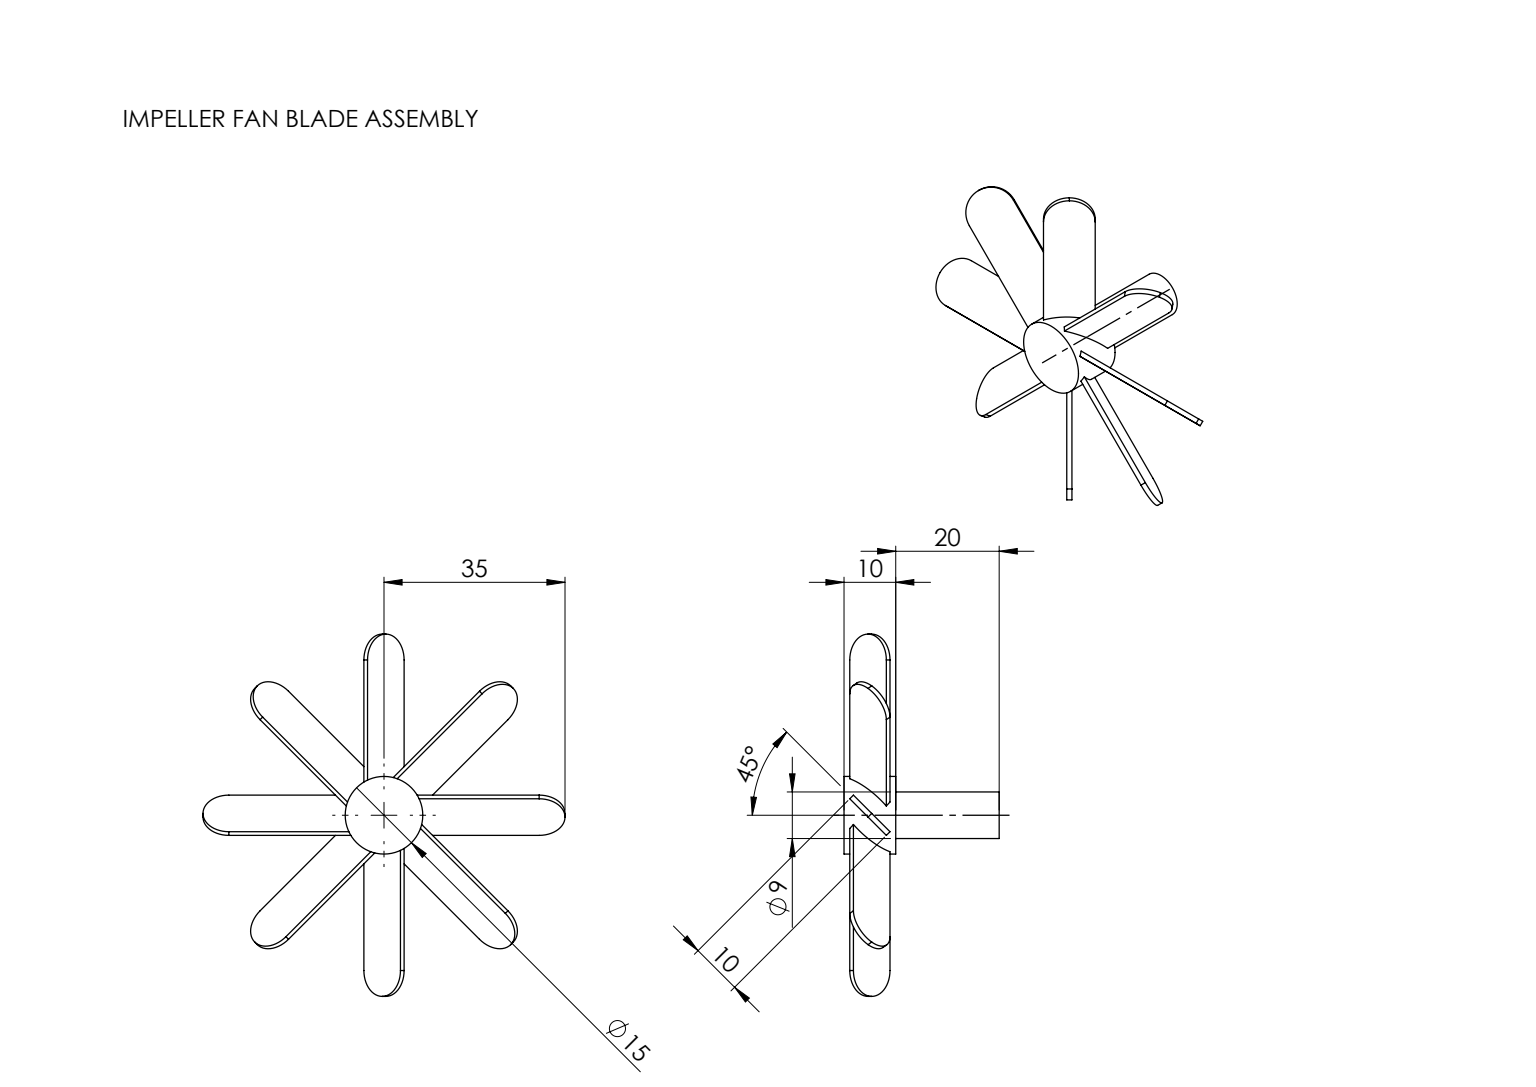
ISO-10303-21;
HEADER;
FILE_DESCRIPTION (('STEP AP214'),
    '1' );
FILE_NAME ('Impeller Fan Blade Assembly.step',
    '2026-10-04T13:31:42',
    ( '' ),
    ( '' ),
    'SwSTEP 2.0',
    'SolidWorks 2026',
    '' );
FILE_SCHEMA (( 'AUTOMOTIVE_DESIGN' ));
ENDSEC;

DATA;
#5=ORIENTED_EDGE ( 'NONE', *, *, #6876, .T. ) ;
#55=EDGE_CURVE ( 'NONE', #141361, #196966, #36036, .T. ) ;
#108=DIRECTION ( 'NONE',  ( -0.000000000000000000, -0.000000000000000000, -1.000000000000000000 ) ) ;
#589=CARTESIAN_POINT ( 'NONE',  ( -30.00000000000000355, 0.3535533905932703447, 5.353553390593268624 ) ) ;
#689=CARTESIAN_POINT ( 'NONE',  ( -3.181980515339399851, 6.791538853603101167, 8.889087296526001936 ) ) ;
#723=VERTEX_POINT ( 'NONE', #107411 ) ;
#910=CIRCLE ( 'NONE', #26805, 5.000000000000000000 ) ;
#1107=EDGE_CURVE ( 'NONE', #17186, #144635, #184276, .T. ) ;
#1119=DIRECTION ( 'NONE',  ( -0.8164965809277249242, 0.000000000000000000, 0.5773502691896271743 ) ) ;
#1198=AXIS2_PLACEMENT_3D ( 'NONE', #589, #95589, #143077 ) ;
#1251=( BOUNDED_CURVE ( )  B_SPLINE_CURVE ( 3, ( #125567, #152909, #47741, #154906 ),
 .UNSPECIFIED., .F., .T. ) 
 B_SPLINE_CURVE_WITH_KNOTS ( ( 4, 4 ),
 ( 2.008945357379067431, 2.115944711806982514 ),
 .UNSPECIFIED. ) 
 CURVE ( )  GEOMETRIC_REPRESENTATION_ITEM ( )  RATIONAL_B_SPLINE_CURVE ( ( 1.000000000000000000, 0.9990461557208837329, 0.9990461557208837329, 1.000000000000000000 ) ) 
 REPRESENTATION_ITEM ( '' )  );
#1322=FACE_OUTER_BOUND ( 'NONE', #192429, .T. ) ;
#1347=EDGE_CURVE ( 'NONE', #15917, #80087, #46585, .T. ) ;
#1367=CARTESIAN_POINT ( 'NONE',  ( 0.3535533905935857035, 30.00000000000000000, 5.353553390593269512 ) ) ;
#1528=CARTESIAN_POINT ( 'NONE',  ( 26.99873734152944138, 22.49873734152883387, 1.110912703473986074 ) ) ;
#1540=CIRCLE ( 'NONE', #59712, 5.000000000000000888 ) ;
#1624=AXIS2_PLACEMENT_3D ( 'NONE', #95423, #190434, #66079 ) ;
#1785=CARTESIAN_POINT ( 'NONE',  ( 4.500000000000000000, 0.000000000000000000, 0.000000000000000000 ) ) ;
#1856=ORIENTED_EDGE ( 'NONE', *, *, #13659, .T. ) ;
#1902=ORIENTED_EDGE ( 'NONE', *, *, #135350, .T. ) ;
#2136=DIRECTION ( 'NONE',  ( -0.7071067811865466846, 2.468850131082262583E-15, 0.7071067811865484609 ) ) ;
#2501=EDGE_CURVE ( 'NONE', #144635, #114656, #107792, .T. ) ;
#2531=DIRECTION ( 'NONE',  ( -0.7071067811865467956, 2.468850131082262977E-15, 0.7071067811865483499 ) ) ;
#2575=ADVANCED_FACE ( 'NONE', ( #39541 ), #193239, .T. ) ;
#2692=CARTESIAN_POINT ( 'NONE',  ( -3.660253528765552655, 6.551653823223177575, 8.410814283099849575 ) ) ;
#2908=DIRECTION ( 'NONE',  ( 0.8164965809277261455, 0.000000000000000000, 0.5773502691896257311 ) ) ;
#2998=CIRCLE ( 'NONE', #35325, 5.000000000000000000 ) ;
#3003=EDGE_CURVE ( 'NONE', #196688, #171715, #100113, .T. ) ;
#3105=EDGE_CURVE ( 'NONE', #165429, #128792, #7889, .T. ) ;
#3150=EDGE_CURVE ( 'NONE', #42832, #9747, #47569, .T. ) ;
#3534=FACE_OUTER_BOUND ( 'NONE', #60688, .T. ) ;
#3693=CARTESIAN_POINT ( 'NONE',  ( -21.99873734152892268, 27.49873734152935967, 1.818019484660534424 ) ) ;
#3699=LINE ( 'NONE', #80542, #50035 ) ;
#3706=CARTESIAN_POINT ( 'NONE',  ( 3.181980515339348337, -35.00000000000001421, 8.889087296526001936 ) ) ;
#3913=CARTESIAN_POINT ( 'NONE',  ( -7.500000000000000888, 1.380023386739105407, 4.327083394447439169 ) ) ;
#3974=PLANE ( 'NONE',  #72309 ) ;
#3984=DIRECTION ( 'NONE',  ( -0.7071067811865467956, 0.000000000000000000, 0.7071067811865483499 ) ) ;
#4050=DIRECTION ( 'NONE',  ( -1.047444401652940164E-14, -1.000000000000000000, -0.000000000000000000 ) ) ;
#4144=CARTESIAN_POINT ( 'NONE',  ( -6.412877669190335972, 3.889087296526014814, 1.818019484660534424 ) ) ;
#4246=VERTEX_POINT ( 'NONE', #76836 ) ;
#4281=CARTESIAN_POINT ( 'NONE',  ( -0.3535533905933930798, -35.00000000000000000, 5.353553390593270400 ) ) ;
#4343=CARTESIAN_POINT ( 'NONE',  ( -30.00000000000000355, 0.3535533905932729537, 5.353553390593267736 ) ) ;
#4363=CIRCLE ( 'NONE', #120577, 4.500000000000000000 ) ;
#4390=EDGE_LOOP ( 'NONE', ( #44839, #29813, #144030, #184763 ) ) ;
#4454=EDGE_CURVE ( 'NONE', #48994, #85047, #178636, .T. ) ;
#4626=VERTEX_POINT ( 'NONE', #89603 ) ;
#4692=ORIENTED_EDGE ( 'NONE', *, *, #3003, .F. ) ;
#4756=DIRECTION ( 'NONE',  ( -0.4999999999999967804, 0.5000000000000019984, 0.7071067811865484609 ) ) ;
#4830=VECTOR ( 'NONE', #8942, 1000.000000000000000 ) ;
#4878=VECTOR ( 'NONE', #141249, 1000.000000000000000 ) ;
#4970=FACE_OUTER_BOUND ( 'NONE', #19771, .T. ) ;
#5025=DIRECTION ( 'NONE',  ( -0.7071067811865466846, 7.406550393246786959E-15, -0.7071067811865484609 ) ) ;
#5159=DIRECTION ( 'NONE',  ( 0.5000000000000004441, 0.4999999999999987232, -0.7071067811865482389 ) ) ;
#5238=CARTESIAN_POINT ( 'NONE',  ( 3.660253528765602393, -6.551653823223149153, 8.410814283099844246 ) ) ;
#5316=CARTESIAN_POINT ( 'NONE',  ( 2.044528755335677683, -7.220908937440018605, 1.589185716900141321 ) ) ;
#5451=ORIENTED_EDGE ( 'NONE', *, *, #13659, .F. ) ;
#5503=CARTESIAN_POINT ( 'NONE',  ( 3.181980515339782212, 29.99999999999996803, 1.110912703473986074 ) ) ;
#5513=DIRECTION ( 'NONE',  ( 0.7071067811865414665, -0.7071067811865536790, -0.000000000000000000 ) ) ;
#5740=CARTESIAN_POINT ( 'NONE',  ( -21.99873734152930638, -27.49873734152905413, 8.181980515339454030 ) ) ;
#5918=CARTESIAN_POINT ( 'NONE',  ( -6.791538853603066528, 3.181980515339468241, 1.110912703473986074 ) ) ;
#5983=ORIENTED_EDGE ( 'NONE', *, *, #3150, .T. ) ;
#6136=AXIS2_PLACEMENT_3D ( 'NONE', #66629, #172837, #37289 ) ;
#6324=CARTESIAN_POINT ( 'NONE',  ( 35.00000000000000000, -3.181980515339468241, 1.110912703473986074 ) ) ;
#6392=ORIENTED_EDGE ( 'NONE', *, *, #134059, .T. ) ;
#6445=ORIENTED_EDGE ( 'NONE', *, *, #56848, .T. ) ;
#6595=VECTOR ( 'NONE', #69761, 1000.000000000000000 ) ;
#6659=CARTESIAN_POINT ( 'NONE',  ( -23.96320343559627375, 18.46320343559663257, 8.181980515339452253 ) ) ;
#6681=VERTEX_POINT ( 'NONE', #26746 ) ;
#6876=EDGE_CURVE ( 'NONE', #157949, #129810, #101294, .T. ) ;
#6906=EDGE_CURVE ( 'NONE', #84463, #144635, #114277, .T. ) ;
#7056=CARTESIAN_POINT ( 'NONE',  ( -3.181980515339590365, -34.99999999999999289, 1.110912703473986074 ) ) ;
#7236=CARTESIAN_POINT ( 'NONE',  ( 3.889087296525994830, -6.412877669190346630, 8.181980515339454030 ) ) ;
#7349=ADVANCED_FACE ( 'NONE', ( #109514 ), #171196, .T. ) ;
#7427=DIRECTION ( 'NONE',  ( 0.7071067811865483499, 0.000000000000000000, -0.7071067811865465735 ) ) ;
#7479=ORIENTED_EDGE ( 'NONE', *, *, #86511, .F. ) ;
#7567=CARTESIAN_POINT ( 'NONE',  ( 3.181980515339834614, 34.99999999999997158, 1.110912703473986074 ) ) ;
#7576=ORIENTED_EDGE ( 'NONE', *, *, #27260, .F. ) ;
#7667=LINE ( 'NONE', #113841, #95061 ) ;
#7672=PLANE ( 'NONE',  #93602 ) ;
#7889=CIRCLE ( 'NONE', #130564, 5.000000000000000000 ) ;
#7900=STYLED_ITEM ( 'NONE', ( #152730 ), #117169 ) ;
#8055=ORIENTED_EDGE ( 'NONE', *, *, #1107, .F. ) ;
#8138=EDGE_CURVE ( 'NONE', #13627, #4626, #1540, .T. ) ;
#8335=SHAPE_REPRESENTATION ( 'Impeller Fan Blade Assembly', ( #82054 ), #65912 ) ;
#8564=DIRECTION ( 'NONE',  ( 0.000000000000000000, -0.7071067811865483499, -0.7071067811865467956 ) ) ;
#8687=CARTESIAN_POINT ( 'NONE',  ( -30.00000000000000355, -0.3535533905932729537, 4.646446609406719830 ) ) ;
#8817=CIRCLE ( 'NONE', #41014, 4.999999999999999112 ) ;
#8942=DIRECTION ( 'NONE',  ( -0.7071067811865561215, -0.7071067811865389130, -0.000000000000000000 ) ) ;
#8948=ADVANCED_FACE ( 'NONE', ( #56337 ), #72517, .T. ) ;
#9057=CARTESIAN_POINT ( 'NONE',  ( 1.784589286804253661, -7.284589286804279418, 1.818019484660534424 ) ) ;
#9330=CARTESIAN_POINT ( 'NONE',  ( 4.500000000000000000, 0.000000000000000000, -20.00000000000000000 ) ) ;
#9490=DIRECTION ( 'NONE',  ( -0.7071067811865483499, 7.406550393246807469E-15, 0.7071067811865467956 ) ) ;
#9504=DIRECTION ( 'NONE',  ( -0.4999999999999966693, 0.5000000000000019984, 0.7071067811865484609 ) ) ;
#9508=VERTEX_POINT ( 'NONE', #142115 ) ;
#9572=CARTESIAN_POINT ( 'NONE',  ( 20.96320343559639454, -21.46320343559646560, 5.353553390593268624 ) ) ;
#9574=CARTESIAN_POINT ( 'NONE',  ( 6.791538853603070081, -3.181980515339468241, 1.110912703473986074 ) ) ;
#9721=ORIENTED_EDGE ( 'NONE', *, *, #167487, .T. ) ;
#9747=VERTEX_POINT ( 'NONE', #90410 ) ;
#10026=CARTESIAN_POINT ( 'NONE',  ( 7.500000000000000000, 9.184850993605147944E-16, 10.00000000000000000 ) ) ;
#10163=DIRECTION ( 'NONE',  ( 3.491481338843133750E-15, 1.000000000000000000, -0.000000000000000000 ) ) ;
#10280=EDGE_CURVE ( 'NONE', #27947, #199067, #69380, .T. ) ;
#10292=AXIS2_PLACEMENT_3D ( 'NONE', #91072, #108246, #169925 ) ;
#10463=DIRECTION ( 'NONE',  ( 3.491481338843133750E-15, 1.000000000000000000, -0.000000000000000000 ) ) ;
#10721=EDGE_LOOP ( 'NONE', ( #25511, #113334, #196537, #77150 ) ) ;
#10785=DIRECTION ( 'NONE',  ( -0.5000000000000004441, -0.4999999999999986122, 0.7071067811865481278 ) ) ;
#10842=EDGE_CURVE ( 'NONE', #178298, #133752, #105049, .T. ) ;
#11040=ORIENTED_EDGE ( 'NONE', *, *, #91376, .T. ) ;
#11092=CIRCLE ( 'NONE', #108041, 5.000000000000000888 ) ;
#11219=ADVANCED_FACE ( 'NONE', ( #166041 ), #39684, .T. ) ;
#11295=DIRECTION ( 'NONE',  ( 0.000000000000000000, 0.000000000000000000, -1.000000000000000000 ) ) ;
#11355=LINE ( 'NONE', #146847, #59682 ) ;
#11514=PLANE ( 'NONE',  #138109 ) ;
#11543=EDGE_LOOP ( 'NONE', ( #139060, #54030, #101271, #76583, #175395 ) ) ;
#11617=ORIENTED_EDGE ( 'NONE', *, *, #69929, .F. ) ;
#11630=AXIS2_PLACEMENT_3D ( 'NONE', #120508, #167033, #180236 ) ;
#11743=CARTESIAN_POINT ( 'NONE',  ( 1.784589286804354247, 7.284589286804251884, 8.181980515339454030 ) ) ;
#11932=( BOUNDED_CURVE ( )  B_SPLINE_CURVE ( 3, ( #178851, #190018, #191005, #82807 ),
 .UNSPECIFIED., .F., .T. ) 
 B_SPLINE_CURVE_WITH_KNOTS ( ( 4, 4 ),
 ( 1.570796326794896780, 2.008945357379067875 ),
 .UNSPECIFIED. ) 
 CURVE ( )  GEOMETRIC_REPRESENTATION_ITEM ( )  RATIONAL_B_SPLINE_CURVE ( ( 1.000000000000000000, 0.9840659996946589105, 0.9840659996946589105, 1.000000000000000000 ) ) 
 REPRESENTATION_ITEM ( '' )  );
#12043=ORIENTED_EDGE ( 'NONE', *, *, #15456, .T. ) ;
#12294=DIRECTION ( 'NONE',  ( 0.7071067811865483499, 0.000000000000000000, 0.7071067811865465735 ) ) ;
#12421=ORIENTED_EDGE ( 'NONE', *, *, #88897, .T. ) ;
#12432=EDGE_CURVE ( 'NONE', #166399, #177515, #11092, .T. ) ;
#12454=LINE ( 'NONE', #42781, #99287 ) ;
#12531=EDGE_LOOP ( 'NONE', ( #95723, #112577, #18902, #136968, #137957 ) ) ;
#12569=CARTESIAN_POINT ( 'NONE',  ( 3.889087296526082316, 6.412877669190294228, 1.818019484660534424 ) ) ;
#12967=ADVANCED_FACE ( 'NONE', ( #39608 ), #101267, .T. ) ;
#13016=EDGE_LOOP ( 'NONE', ( #106007, #37558 ) ) ;
#13023=EDGE_LOOP ( 'NONE', ( #163707, #150234, #31137, #136726 ) ) ;
#13033=ORIENTED_EDGE ( 'NONE', *, *, #147612, .T. ) ;
#13111=EDGE_CURVE ( 'NONE', #198713, #191800, #40221, .T. ) ;
#13247=SURFACE_SIDE_STYLE ('',( #59729 ) ) ;
#13272=CARTESIAN_POINT ( 'NONE',  ( -0.3535533905933784249, -30.00000000000000000, 5.353553390593268624 ) ) ;
#13320=EDGE_CURVE ( 'NONE', #81477, #29557, #156408, .T. ) ;
#13428=CARTESIAN_POINT ( 'NONE',  ( -3.889087296526120063, -29.99999999999998579, 1.818019484660534424 ) ) ;
#13627=VERTEX_POINT ( 'NONE', #119460 ) ;
#13659=EDGE_CURVE ( 'NONE', #42657, #30159, #117744, .T. ) ;
#13686=EDGE_LOOP ( 'NONE', ( #100957, #99162, #122870, #78497, #107366, #112026 ) ) ;
#13931=CARTESIAN_POINT ( 'NONE',  ( -2.044528755335630166, 7.220908937440031039, 1.589185716900140211 ) ) ;
#14009=CARTESIAN_POINT ( 'NONE',  ( -18.46320343559655086, -23.96320343559633059, 8.181980515339455806 ) ) ;
#14059=LINE ( 'NONE', #26274, #159692 ) ;
#14195=EDGE_CURVE ( 'NONE', #96881, #9508, #7667, .T. ) ;
#14313=VECTOR ( 'NONE', #102691, 1000.000000000000114 ) ;
#14408=DIRECTION ( 'NONE',  ( 0.000000000000000000, 0.7071067811865467956, -0.7071067811865483499 ) ) ;
#14414=LINE ( 'NONE', #123563, #33888 ) ;
#14524=CIRCLE ( 'NONE', #82328, 5.000000000000000888 ) ;
#14739=CARTESIAN_POINT ( 'NONE',  ( -7.220908937440027486, -2.044528755335643044, 1.589185716900149092 ) ) ;
#14812=ORIENTED_EDGE ( 'NONE', *, *, #128355, .F. ) ;
#14925=DIRECTION ( 'NONE',  ( 0.5000000000000037748, 0.4999999999999950595, 0.7071067811865484609 ) ) ;
#15121=CARTESIAN_POINT ( 'NONE',  ( -30.00000000000000355, -3.889087296526017479, 8.181980515339454030 ) ) ;
#15152=VECTOR ( 'NONE', #148657, 1000.000000000000000 ) ;
#15282=VECTOR ( 'NONE', #95551, 1000.000000000000000 ) ;
#15456=EDGE_CURVE ( 'NONE', #9747, #199879, #95459, .T. ) ;
#15553=CARTESIAN_POINT ( 'NONE',  ( 30.00000000000000355, -3.889087296526015258, 1.818019484660534646 ) ) ;
#15917=VERTEX_POINT ( 'NONE', #99441 ) ;
#15975=CIRCLE ( 'NONE', #116131, 5.000000000000000000 ) ;
#16098=LINE ( 'NONE', #64586, #153351 ) ;
#16296=DIRECTION ( 'NONE',  ( -1.000000000000000000, 0.000000000000000000, 0.000000000000000000 ) ) ;
#16411=CARTESIAN_POINT ( 'NONE',  ( -2.552343178074661267, -7.052343178074616858, 8.889087296526001936 ) ) ;
#16715=DIRECTION ( 'NONE',  ( 0.5000000000000014433, 0.4999999999999996114, 0.7071067811865467956 ) ) ;
#16726=CARTESIAN_POINT ( 'NONE',  ( 6.791538853603062975, 3.181980515339470905, 8.889087296526001936 ) ) ;
#16796=ORIENTED_EDGE ( 'NONE', *, *, #105651, .T. ) ;
#16838=EDGE_CURVE ( 'NONE', #172390, #19226, #143704, .T. ) ;
#16899=CARTESIAN_POINT ( 'NONE',  ( 6.412877669190335972, -3.889087296526014814, 1.818019484660534424 ) ) ;
#17186=VERTEX_POINT ( 'NONE', #124573 ) ;
#17220=ORIENTED_EDGE ( 'NONE', *, *, #112155, .T. ) ;
#17363=VERTEX_POINT ( 'NONE', #16411 ) ;
#17418=EDGE_CURVE ( 'NONE', #75343, #15917, #153385, .T. ) ;
#17615=EDGE_CURVE ( 'NONE', #85047, #60651, #14414, .T. ) ;
#17635=DIRECTION ( 'NONE',  ( -0.000000000000000000, -0.000000000000000000, -1.000000000000000000 ) ) ;
#17870=AXIS2_PLACEMENT_3D ( 'NONE', #4343, #130687, #157056 ) ;
#17909=ORIENTED_EDGE ( 'NONE', *, *, #89293, .T. ) ;
#17930=DIRECTION ( 'NONE',  ( 0.000000000000000000, -0.7071067811865467956, -0.7071067811865483499 ) ) ;
#18096=CARTESIAN_POINT ( 'NONE',  ( -7.284589286804255437, 1.784589286804319386, 8.181980515339454030 ) ) ;
#18224=VERTEX_POINT ( 'NONE', #160889 ) ;
#18467=VECTOR ( 'NONE', #74443, 1000.000000000000000 ) ;
#18598=ORIENTED_EDGE ( 'NONE', *, *, #48667, .F. ) ;
#18660=ORIENTED_EDGE ( 'NONE', *, *, #193497, .T. ) ;
#18750=AXIS2_PLACEMENT_3D ( 'NONE', #120314, #42501, #61612 ) ;
#18902=ORIENTED_EDGE ( 'NONE', *, *, #136231, .T. ) ;
#18906=EDGE_CURVE ( 'NONE', #96881, #27352, #98517, .T. ) ;
#19107=CARTESIAN_POINT ( 'NONE',  ( -7.128481858827110607, 2.709097808555396281, 2.998008972631150737 ) ) ;
#19109=DIRECTION ( 'NONE',  ( 0.7071067811865483499, -2.468850131082268499E-15, 0.7071067811865467956 ) ) ;
#19226=VERTEX_POINT ( 'NONE', #185021 ) ;
#19309=CARTESIAN_POINT ( 'NONE',  ( -3.181980515339399851, 6.791538853603101167, 8.889087296526001936 ) ) ;
#19710=DIRECTION ( 'NONE',  ( 0.000000000000000000, -0.8164965809277239250, -0.5773502691896288397 ) ) ;
#19771=EDGE_LOOP ( 'NONE', ( #190197, #68449, #74086, #157970 ) ) ;
#19850=CARTESIAN_POINT ( 'NONE',  ( -3.424326230466266718, 6.677994727576254341, 8.646741581399135512 ) ) ;
#19925=ADVANCED_FACE ( 'NONE', ( #188018 ), #156674, .T. ) ;
#19960=EDGE_LOOP ( 'NONE', ( #159693, #6392, #38372, #30787 ) ) ;
#20100=PLANE ( 'NONE',  #147708 ) ;
#20134=CARTESIAN_POINT ( 'NONE',  ( 0.3535533905935844268, 30.00000000000000000, 5.353553390593268624 ) ) ;
#20188=ORIENTED_EDGE ( 'NONE', *, *, #57355, .T. ) ;
#20191=DIRECTION ( 'NONE',  ( -0.4999999999999966693, 0.5000000000000019984, 0.7071067811865483499 ) ) ;
#20248=EDGE_CURVE ( 'NONE', #178298, #138583, #149478, .T. ) ;
#20336=DIRECTION ( 'NONE',  ( 0.5000000000000037748, 0.4999999999999950040, 0.7071067811865484609 ) ) ;
#20570=VERTEX_POINT ( 'NONE', #197973 ) ;
#20607=DIRECTION ( 'NONE',  ( 1.000000000000000000, 0.000000000000000000, -0.000000000000000000 ) ) ;
#20686=ORIENTED_EDGE ( 'NONE', *, *, #10842, .T. ) ;
#20694=CARTESIAN_POINT ( 'NONE',  ( -22.49873734152930282, -26.99873734152905058, 8.889087296526001936 ) ) ;
#20858=CARTESIAN_POINT ( 'NONE',  ( 3.181980515339539295, 6.791538853603031889, 1.110912703473986074 ) ) ;
#20991=VECTOR ( 'NONE', #68552, 1000.000000000000000 ) ;
#21095=CARTESIAN_POINT ( 'NONE',  ( -7.500000000000000000, 0.000000000000000000, 4.292893218813445877 ) ) ;
#21117=LINE ( 'NONE', #174809, #43151 ) ;
#21147=VECTOR ( 'NONE', #98013, 1000.000000000000000 ) ;
#21379=DIRECTION ( 'NONE',  ( 0.000000000000000000, 0.8164965809277239250, 0.5773502691896288397 ) ) ;
#21384=VECTOR ( 'NONE', #104477, 1000.000000000000000 ) ;
#21394=ORIENTED_EDGE ( 'NONE', *, *, #126396, .T. ) ;
#21707=CARTESIAN_POINT ( 'NONE',  ( 27.49873734152913229, -21.99873734152921045, 8.181980515339454030 ) ) ;
#21733=FACE_OUTER_BOUND ( 'NONE', #88711, .T. ) ;
#21856=DIRECTION ( 'NONE',  ( 1.000000000000000000, -0.000000000000000000, -0.000000000000000000 ) ) ;
#22083=CARTESIAN_POINT ( 'NONE',  ( -6.412877669190335972, 3.889087296526014814, 1.818019484660534424 ) ) ;
#22192=ORIENTED_EDGE ( 'NONE', *, *, #13320, .T. ) ;
#22226=DIRECTION ( 'NONE',  ( 1.000000000000000000, -0.000000000000000000, -0.000000000000000000 ) ) ;
#22425=CARTESIAN_POINT ( 'NONE',  ( 3.181980515339446924, -6.791538853603077186, 8.889087296526001936 ) ) ;
#22619=PLANE ( 'NONE',  #91802 ) ;
#22670=EDGE_LOOP ( 'NONE', ( #127996, #170160, #88143, #37570 ) ) ;
#22862=CARTESIAN_POINT ( 'NONE',  ( -22.49873734152892624, 26.99873734152936677, 1.110912703473986074 ) ) ;
#22871=DIRECTION ( 'NONE',  ( -0.5000000000000037748, -0.4999999999999950595, -0.7071067811865484609 ) ) ;
#23387=CARTESIAN_POINT ( 'NONE',  ( -7.500000000000000000, 0.000000000000000000, 5.707106781186540800 ) ) ;
#23431=ORIENTED_EDGE ( 'NONE', *, *, #100813, .F. ) ;
#23455=ORIENTED_EDGE ( 'NONE', *, *, #67374, .T. ) ;
#23492=DIRECTION ( 'NONE',  ( -0.5000000000000037748, -0.4999999999999950595, -0.7071067811865484609 ) ) ;
#23611=VERTEX_POINT ( 'NONE', #176579 ) ;
#23632=CARTESIAN_POINT ( 'NONE',  ( -7.052343178074620411, 2.552343178074692354, 8.889087296526001936 ) ) ;
#23740=CARTESIAN_POINT ( 'NONE',  ( 3.660253528765689435, 6.551653823223101192, 1.589185716900141543 ) ) ;
#23852=DIRECTION ( 'NONE',  ( -0.000000000000000000, 0.7071067811865466846, -0.7071067811865484609 ) ) ;
#23886=AXIS2_PLACEMENT_3D ( 'NONE', #181840, #166675, #55488 ) ;
#24008=ORIENTED_EDGE ( 'NONE', *, *, #133545, .T. ) ;
#24394=DIRECTION ( 'NONE',  ( 0.000000000000000000, -0.7071067811865485719, 0.7071067811865465735 ) ) ;
#24399=CARTESIAN_POINT ( 'NONE',  ( -26.99873734152928506, -22.49873734152901861, 1.110912703473986074 ) ) ;
#24590=ORIENTED_EDGE ( 'NONE', *, *, #123454, .T. ) ;
#24593=ORIENTED_EDGE ( 'NONE', *, *, #170916, .F. ) ;
#24595=ORIENTED_EDGE ( 'NONE', *, *, #145326, .F. ) ;
#24627=CARTESIAN_POINT ( 'NONE',  ( 21.99873734152949822, 27.49873734152890137, 8.181980515339454030 ) ) ;
#24679=CYLINDRICAL_SURFACE ( 'NONE', #186623, 5.000000000000002665 ) ;
#24832=ORIENTED_EDGE ( 'NONE', *, *, #149135, .T. ) ;
#25131=ORIENTED_EDGE ( 'NONE', *, *, #52643, .F. ) ;
#25203=CARTESIAN_POINT ( 'NONE',  ( 20.96320343559668942, 21.46320343559617427, 4.646446609406718942 ) ) ;
#25449=EDGE_CURVE ( 'NONE', #144525, #33153, #188245, .T. ) ;
#25474=CARTESIAN_POINT ( 'NONE',  ( 0.000000000000000000, 0.000000000000000000, 0.000000000000000000 ) ) ;
#25511=ORIENTED_EDGE ( 'NONE', *, *, #129609, .F. ) ;
#25535=CARTESIAN_POINT ( 'NONE',  ( 2.552343178074723884, 7.052343178074616858, 8.889087296526001936 ) ) ;
#25754=CARTESIAN_POINT ( 'NONE',  ( 6.551653823223139383, -3.660253528765621045, 1.589185716900141543 ) ) ;
#25888=ORIENTED_EDGE ( 'NONE', *, *, #28343, .F. ) ;
#26096=( BOUNDED_CURVE ( )  B_SPLINE_CURVE ( 3, ( #116778, #194637, #103622, #42945 ),
 .UNSPECIFIED., .F., .T. ) 
 B_SPLINE_CURVE_WITH_KNOTS ( ( 4, 4 ),
 ( 1.132647296210726795, 2.115944711806982514 ),
 .UNSPECIFIED. ) 
 CURVE ( )  GEOMETRIC_REPRESENTATION_ITEM ( )  RATIONAL_B_SPLINE_CURVE ( ( 1.000000000000000000, 0.9210371567966664230, 0.9210371567966664230, 1.000000000000000000 ) ) 
 REPRESENTATION_ITEM ( '' )  );
#26126=VERTEX_POINT ( 'NONE', #40621 ) ;
#26274=CARTESIAN_POINT ( 'NONE',  ( 3.889087296525912674, -30.00000000000002132, 8.181980515339454030 ) ) ;
#26660=CARTESIAN_POINT ( 'NONE',  ( -3.181980515339104532, 35.00000000000003553, 8.889087296526001936 ) ) ;
#26746=CARTESIAN_POINT ( 'NONE',  ( -30.00000000000000355, -3.181980515339470905, 8.889087296526001936 ) ) ;
#26791=CARTESIAN_POINT ( 'NONE',  ( 3.889087296526381632, 34.99999999999996447, 1.818019484660534424 ) ) ;
#26805=AXIS2_PLACEMENT_3D ( 'NONE', #91589, #92593, #153279 ) ;
#26877=CARTESIAN_POINT ( 'NONE',  ( -4.500000000000000000, 5.510910596163088569E-16, -20.00000000000000000 ) ) ;
#26894=VERTEX_POINT ( 'NONE', #49568 ) ;
#27082=AXIS2_PLACEMENT_3D ( 'NONE', #20694, #84353, #19710 ) ;
#27260=EDGE_CURVE ( 'NONE', #90645, #95772, #139430, .T. ) ;
#27280=MECHANICAL_DESIGN_GEOMETRIC_PRESENTATION_REPRESENTATION('',(#7900),#130572);
#27352=VERTEX_POINT ( 'NONE', #184110 ) ;
#27375=ORIENTED_EDGE ( 'NONE', *, *, #136231, .F. ) ;
#27439=EDGE_LOOP ( 'NONE', ( #5, #177531, #143908, #11617 ) ) ;
#27493=AXIS2_PLACEMENT_3D ( 'NONE', #111358, #20336, #63870 ) ;
#27596=ORIENTED_EDGE ( 'NONE', *, *, #126710, .F. ) ;
#27682=CARTESIAN_POINT ( 'NONE',  ( 21.46320343559668231, 20.96320343559617072, 5.353553390593268624 ) ) ;
#27947=VERTEX_POINT ( 'NONE', #144552 ) ;
#28043=EDGE_CURVE ( 'NONE', #60651, #37524, #38130, .T. ) ;
#28210=ADVANCED_FACE ( 'NONE', ( #138111 ), #87873, .F. ) ;
#28306=VERTEX_POINT ( 'NONE', #162728 ) ;
#28321=CARTESIAN_POINT ( 'NONE',  ( 35.00000000000000000, -0.3535533905932707888, 5.353553390593270400 ) ) ;
#28343=EDGE_CURVE ( 'NONE', #37524, #123075, #155634, .T. ) ;
#28437=VERTEX_POINT ( 'NONE', #85884 ) ;
#28509=CYLINDRICAL_SURFACE ( 'NONE', #190488, 7.500000000000000000 ) ;
#28733=DIRECTION ( 'NONE',  ( -0.5000000000000004441, -0.4999999999999987232, 0.7071067811865482389 ) ) ;
#29121=AXIS2_PLACEMENT_3D ( 'NONE', #119864, #43028, #90504 ) ;
#29203=CARTESIAN_POINT ( 'NONE',  ( 35.00000000000000000, -3.181980515339468241, 1.110912703473986074 ) ) ;
#29290=VECTOR ( 'NONE', #123695, 1000.000000000000000 ) ;
#29437=DIRECTION ( 'NONE',  ( 0.000000000000000000, 0.000000000000000000, -1.000000000000000000 ) ) ;
#29441=EDGE_LOOP ( 'NONE', ( #71166, #121903, #199643, #195876, #16796, #178830 ) ) ;
#29557=VERTEX_POINT ( 'NONE', #181399 ) ;
#29584=CARTESIAN_POINT ( 'NONE',  ( -6.791538853603066528, -3.181980515339470905, 8.889087296526001936 ) ) ;
#29707=DIRECTION ( 'NONE',  ( -0.000000000000000000, -0.7071067811865467956, 0.7071067811865483499 ) ) ;
#29813=ORIENTED_EDGE ( 'NONE', *, *, #165696, .T. ) ;
#30159=VERTEX_POINT ( 'NONE', #4281 ) ;
#30610=CYLINDRICAL_SURFACE ( 'NONE', #50415, 5.000000000000000000 ) ;
#30636=VERTEX_POINT ( 'NONE', #44613 ) ;
#30664=ORIENTED_EDGE ( 'NONE', *, *, #41288, .F. ) ;
#30694=DIRECTION ( 'NONE',  ( 0.000000000000000000, -0.7071067811865467956, 0.7071067811865483499 ) ) ;
#30703=CARTESIAN_POINT ( 'NONE',  ( 24.49873734152946625, 24.99873734152886939, 4.646446609406719830 ) ) ;
#30787=ORIENTED_EDGE ( 'NONE', *, *, #94101, .F. ) ;
#30940=CARTESIAN_POINT ( 'NONE',  ( 7.143419655154867876, -2.300691058039452397, 8.646741581399133736 ) ) ;
#30966=FACE_OUTER_BOUND ( 'NONE', #4390, .T. ) ;
#31031=AXIS2_PLACEMENT_3D ( 'NONE', #198438, #165127, #58921 ) ;
#31085=ORIENTED_EDGE ( 'NONE', *, *, #135350, .F. ) ;
#31137=ORIENTED_EDGE ( 'NONE', *, *, #28343, .T. ) ;
#31165=DIRECTION ( 'NONE',  ( 0.000000000000000000, 0.000000000000000000, 1.000000000000000000 ) ) ;
#31316=VECTOR ( 'NONE', #88433, 1000.000000000000000 ) ;
#31365=DIRECTION ( 'NONE',  ( -0.7071067811865483499, 2.468850131082268499E-15, -0.7071067811865467956 ) ) ;
#31456=EDGE_CURVE ( 'NONE', #199067, #20570, #94075, .T. ) ;
#31479=PLANE ( 'NONE',  #192537 ) ;
#31687=CARTESIAN_POINT ( 'NONE',  ( 0.3535533905935877019, 30.00000000000000000, 5.353553390593268624 ) ) ;
#31691=CARTESIAN_POINT ( 'NONE',  ( 7.500000000000000000, 9.184850993605147944E-16, 5.707106781186540800 ) ) ;
#31820=EDGE_CURVE ( 'NONE', #6681, #171715, #66728, .T. ) ;
#31887=DIRECTION ( 'NONE',  ( 0.7071067811865483499, 0.000000000000000000, 0.7071067811865465735 ) ) ;
#31995=VECTOR ( 'NONE', #149468, 1000.000000000000114 ) ;
#32158=CARTESIAN_POINT ( 'NONE',  ( 2.552343178074723884, 7.052343178074616858, 8.889087296526001936 ) ) ;
#32252=ORIENTED_EDGE ( 'NONE', *, *, #73850, .T. ) ;
#32283=CARTESIAN_POINT ( 'NONE',  ( 27.49873734152943427, 21.99873734152882676, 1.818019484660534424 ) ) ;
#32299=ORIENTED_EDGE ( 'NONE', *, *, #185673, .F. ) ;
#32314=AXIS2_PLACEMENT_3D ( 'NONE', #108190, #31365, #3984 ) ;
#33093=FACE_OUTER_BOUND ( 'NONE', #180286, .T. ) ;
#33146=ORIENTED_EDGE ( 'NONE', *, *, #177829, .F. ) ;
#33153=VERTEX_POINT ( 'NONE', #133397 ) ;
#33338=DIRECTION ( 'NONE',  ( -0.4999999999999932832, 0.5000000000000055511, -0.7071067811865483499 ) ) ;
#33560=ADVANCED_FACE ( 'NONE', ( #30966 ), #63277, .T. ) ;
#33597=VECTOR ( 'NONE', #53965, 1000.000000000000000 ) ;
#33704=VECTOR ( 'NONE', #33338, 1000.000000000000114 ) ;
#33763=FACE_OUTER_BOUND ( 'NONE', #130824, .T. ) ;
#33872=FACE_OUTER_BOUND ( 'NONE', #199222, .T. ) ;
#33881=CARTESIAN_POINT ( 'NONE',  ( -27.49873734152897953, 21.99873734152939875, 8.181980515339454030 ) ) ;
#33888=VECTOR ( 'NONE', #60906, 1000.000000000000000 ) ;
#33943=DIRECTION ( 'NONE',  ( 0.7071067811865485719, -2.775557561562891351E-15, 0.7071067811865465735 ) ) ;
#34033=CARTESIAN_POINT ( 'NONE',  ( -3.889087296525950421, 6.412877669190374164, 8.181980515339454030 ) ) ;
#34239=ORIENTED_EDGE ( 'NONE', *, *, #197329, .T. ) ;
#34333=FACE_OUTER_BOUND ( 'NONE', #131122, .T. ) ;
#34450=ADVANCED_FACE ( 'NONE', ( #123694, #93363, #198588, #108543 ), #44900, .T. ) ;
#34761=ORIENTED_EDGE ( 'NONE', *, *, #69929, .T. ) ;
#34781=DIRECTION ( 'NONE',  ( -1.047444401652940164E-14, -1.000000000000000000, -0.000000000000000000 ) ) ;
#35019=CARTESIAN_POINT ( 'NONE',  ( -21.46320343559653665, -20.96320343559631638, 5.353553390593267736 ) ) ;
#35131=ORIENTED_EDGE ( 'NONE', *, *, #12432, .F. ) ;
#35198=CARTESIAN_POINT ( 'NONE',  ( 7.500000000000000000, 9.184850993605147944E-16, 4.292893218813446765 ) ) ;
#35200=LINE ( 'NONE', #65531, #85282 ) ;
#35202=LINE ( 'NONE', #146352, #171004 ) ;
#35260=FACE_OUTER_BOUND ( 'NONE', #88844, .T. ) ;
#35273=CARTESIAN_POINT ( 'NONE',  ( -7.260022482700430047, 2.182060888568184698, 2.110832330245266508 ) ) ;
#35325=AXIS2_PLACEMENT_3D ( 'NONE', #185200, #46691, #78005 ) ;
#35339=EDGE_CURVE ( 'NONE', #723, #84463, #144840, .T. ) ;
#35341=ORIENTED_EDGE ( 'NONE', *, *, #3150, .F. ) ;
#35666=CARTESIAN_POINT ( 'NONE',  ( 1.784589286804253661, -7.284589286804279418, 1.818019484660534424 ) ) ;
#35688=EDGE_CURVE ( 'NONE', #177515, #172390, #11355, .T. ) ;
#35739=EDGE_LOOP ( 'NONE', ( #165093, #7576 ) ) ;
#35745=CARTESIAN_POINT ( 'NONE',  ( -22.49873734152930282, -26.99873734152905058, 8.889087296526001936 ) ) ;
#35780=DIRECTION ( 'NONE',  ( 0.000000000000000000, 0.000000000000000000, 1.000000000000000000 ) ) ;
#35864=PLANE ( 'NONE',  #76338 ) ;
#36010=DIRECTION ( 'NONE',  ( 0.000000000000000000, 0.7071067811865483499, -0.7071067811865466846 ) ) ;
#36019=CARTESIAN_POINT ( 'NONE',  ( -6.180203150055817218, 4.962140900324484960, 6.568406857878972716 ) ) ;
#36023=CARTESIAN_POINT ( 'NONE',  ( 0.8613000766925150709, 7.878827036337479939, 3.431593142121015294 ) ) ;
#36036=LINE ( 'NONE', #3706, #107910 ) ;
#36079=DIRECTION ( 'NONE',  ( 0.7071067811865512365, 0.7071067811865439090, -0.000000000000000000 ) ) ;
#36216=CARTESIAN_POINT ( 'NONE',  ( 7.052343178074640839, -2.552343178074650609, 8.889087296526001936 ) ) ;
#36310=EDGE_CURVE ( 'NONE', #116832, #52906, #117243, .T. ) ;
#36491=ORIENTED_EDGE ( 'NONE', *, *, #122650, .F. ) ;
#36597=CARTESIAN_POINT ( 'NONE',  ( 30.00000000000000355, -0.3535533905932712884, 5.353553390593269512 ) ) ;
#36600=CARTESIAN_POINT ( 'NONE',  ( 0.3535533905931687038, -30.00000000000000355, 4.646446609406718942 ) ) ;
#36780=EDGE_CURVE ( 'NONE', #75343, #116832, #16098, .T. ) ;
#36811=EDGE_CURVE ( 'NONE', #132628, #152161, #72698, .T. ) ;
#36850=FACE_OUTER_BOUND ( 'NONE', #163276, .T. ) ;
#36918=VERTEX_POINT ( 'NONE', #18096 ) ;
#37161=ORIENTED_EDGE ( 'NONE', *, *, #99437, .F. ) ;
#37189=AXIS2_PLACEMENT_3D ( 'NONE', #162885, #164900, #24394 ) ;
#37272=EDGE_CURVE ( 'NONE', #4246, #95772, #128228, .T. ) ;
#37289=DIRECTION ( 'NONE',  ( 1.000000000000000000, 0.000000000000000000, 0.000000000000000000 ) ) ;
#37374=EDGE_CURVE ( 'NONE', #180340, #196688, #84709, .T. ) ;
#37524=VERTEX_POINT ( 'NONE', #36216 ) ;
#37558=ORIENTED_EDGE ( 'NONE', *, *, #147508, .T. ) ;
#37570=ORIENTED_EDGE ( 'NONE', *, *, #6906, .F. ) ;
#37612=VERTEX_POINT ( 'NONE', #54394 ) ;
#37778=DIRECTION ( 'NONE',  ( 0.7071067811865466846, -7.406550393246786959E-15, 0.7071067811865484609 ) ) ;
#37783=CARTESIAN_POINT ( 'NONE',  ( -35.00000000000000000, 3.889087296526014814, 1.818019484660534424 ) ) ;
#37792=VECTOR ( 'NONE', #191542, 1000.000000000000000 ) ;
#37796=UNCERTAINTY_MEASURE_WITH_UNIT (LENGTH_MEASURE( 1.000000000000000082E-05 ), #190273, 'distance_accuracy_value', 'NONE');
#38031=DIRECTION ( 'NONE',  ( 0.5000000000000037748, 0.4999999999999950040, 0.7071067811865483499 ) ) ;
#38130=( BOUNDED_CURVE ( )  B_SPLINE_CURVE ( 3, ( #9057, #103057, #42391, #134405 ),
 .UNSPECIFIED., .F., .T. ) 
 B_SPLINE_CURVE_WITH_KNOTS ( ( 4, 4 ),
 ( 1.025647941782810824, 2.008945357379066987 ),
 .UNSPECIFIED. ) 
 CURVE ( )  GEOMETRIC_REPRESENTATION_ITEM ( )  RATIONAL_B_SPLINE_CURVE ( ( 1.000000000000000000, 0.9210371567966664230, 0.9210371567966664230, 1.000000000000000000 ) ) 
 REPRESENTATION_ITEM ( '' )  );
#38296=LINE ( 'NONE', #39291, #31995 ) ;
#38372=ORIENTED_EDGE ( 'NONE', *, *, #155322, .T. ) ;
#38376=LINE ( 'NONE', #96053, #21147 ) ;
#38554=CARTESIAN_POINT ( 'NONE',  ( 20.96320343559668942, 21.46320343559617427, 4.646446609406719830 ) ) ;
#38588=ADVANCED_FACE ( 'NONE', ( #47105 ), #108765, .T. ) ;
#39044=ORIENTED_EDGE ( 'NONE', *, *, #145326, .T. ) ;
#39096=CARTESIAN_POINT ( 'NONE',  ( 35.00000000000000000, -3.889087296526014814, 1.818019484660534424 ) ) ;
#39291=CARTESIAN_POINT ( 'NONE',  ( 24.99873734152946270, 24.49873734152886229, 5.353553390593268624 ) ) ;
#39319=CARTESIAN_POINT ( 'NONE',  ( 25.54568634023502582, -20.96320343559646915, 7.533197955354848929 ) ) ;
#39349=CARTESIAN_POINT ( 'NONE',  ( 30.00000000000000355, 3.181980515339470905, 8.889087296526001936 ) ) ;
#39358=ORIENTED_EDGE ( 'NONE', *, *, #31820, .F. ) ;
#39541=FACE_OUTER_BOUND ( 'NONE', #150311, .T. ) ;
#39608=FACE_OUTER_BOUND ( 'NONE', #92199, .T. ) ;
#39652=DIRECTION ( 'NONE',  ( 0.4999999999999967248, -0.5000000000000019984, -0.7071067811865484609 ) ) ;
#39684=PLANE ( 'NONE',  #130858 ) ;
#39687=FACE_OUTER_BOUND ( 'NONE', #80548, .T. ) ;
#39897=ADVANCED_FACE ( 'NONE', ( #177317 ), #192469, .T. ) ;
#40003=LINE ( 'NONE', #6659, #82972 ) ;
#40085=AXIS2_PLACEMENT_3D ( 'NONE', #91233, #72124, #195489 ) ;
#40135=ADVANCED_FACE ( 'NONE', ( #161122 ), #22619, .F. ) ;
#40219=EDGE_CURVE ( 'NONE', #86241, #26894, #83557, .T. ) ;
#40221=CIRCLE ( 'NONE', #62725, 4.500000000000000000 ) ;
#40412=AXIS2_PLACEMENT_3D ( 'NONE', #179831, #41301, #55457 ) ;
#40523=CARTESIAN_POINT ( 'NONE',  ( 7.143419655154898962, 2.300691058039359138, 1.353258418600855606 ) ) ;
#40554=DIRECTION ( 'NONE',  ( 0.000000000000000000, -0.8164965809277232589, -0.5773502691896295058 ) ) ;
#40621=CARTESIAN_POINT ( 'NONE',  ( -2.552343178074577779, 7.052343178074668373, 1.110912703473986074 ) ) ;
#40743=ORIENTED_EDGE ( 'NONE', *, *, #8138, .F. ) ;
#41014=AXIS2_PLACEMENT_3D ( 'NONE', #35019, #172548, #64369 ) ;
#41034=DIRECTION ( 'NONE',  ( 0.8164965809277242581, 0.000000000000000000, -0.5773502691896281735 ) ) ;
#41047=AXIS2_PLACEMENT_3D ( 'NONE', #57516, #16715, #119184 ) ;
#41055=ADVANCED_FACE ( 'NONE', ( #85507 ), #147196, .T. ) ;
#41288=EDGE_CURVE ( 'NONE', #152161, #28437, #43019, .T. ) ;
#41301=DIRECTION ( 'NONE',  ( -0.7071067811865466846, 7.406550393246786959E-15, -0.7071067811865484609 ) ) ;
#41499=CARTESIAN_POINT ( 'NONE',  ( 3.889087296525895354, -35.00000000000001421, 8.181980515339454030 ) ) ;
#41517=VERTEX_POINT ( 'NONE', #105672 ) ;
#41598=FILL_AREA_STYLE_COLOUR ( '', #195127 ) ;
#41619=EDGE_CURVE ( 'NONE', #153939, #132628, #118873, .T. ) ;
#41696=DIRECTION ( 'NONE',  ( -0.4999999999999966693, 0.5000000000000018874, 0.7071067811865484609 ) ) ;
#41751=ORIENTED_EDGE ( 'NONE', *, *, #94101, .T. ) ;
#41878=CARTESIAN_POINT ( 'NONE',  ( 7.500000000000000000, 9.184850993605147944E-16, 4.292893218813446765 ) ) ;
#41995=ORIENTED_EDGE ( 'NONE', *, *, #31456, .F. ) ;
#42031=DIRECTION ( 'NONE',  ( -0.5000000000000004441, -0.4999999999999986677, 0.7071067811865481278 ) ) ;
#42144=AXIS2_PLACEMENT_3D ( 'NONE', #98572, #187646, #49117 ) ;
#42187=DIRECTION ( 'NONE',  ( -0.4999999999999933942, 0.5000000000000055511, -0.7071067811865484609 ) ) ;
#42287=ORIENTED_EDGE ( 'NONE', *, *, #160293, .T. ) ;
#42291=CARTESIAN_POINT ( 'NONE',  ( -20.96320343559624177, 21.46320343559660770, 5.353553390593268624 ) ) ;
#42391=CARTESIAN_POINT ( 'NONE',  ( 6.180203150055848305, -4.962140900324442327, 6.568406857878970939 ) ) ;
#42501=DIRECTION ( 'NONE',  ( -0.4999999999999967248, 0.5000000000000019984, 0.7071067811865485719 ) ) ;
#42526=DIRECTION ( 'NONE',  ( 0.4999999999999967248, -0.5000000000000019984, -0.7071067811865485719 ) ) ;
#42569=ORIENTED_EDGE ( 'NONE', *, *, #179632, .T. ) ;
#42622=EDGE_CURVE ( 'NONE', #165429, #58517, #195479, .T. ) ;
#42657=VERTEX_POINT ( 'NONE', #13428 ) ;
#42781=CARTESIAN_POINT ( 'NONE',  ( -3.889087296526120507, -29.99999999999998579, 1.818019484660534868 ) ) ;
#42832=VERTEX_POINT ( 'NONE', #87279 ) ;
#42869=CARTESIAN_POINT ( 'NONE',  ( 7.128481858827108830, 2.709097808555399833, 7.001991027368838161 ) ) ;
#42945=CARTESIAN_POINT ( 'NONE',  ( 1.784589286804354247, 7.284589286804251884, 8.181980515339454030 ) ) ;
#43019=LINE ( 'NONE', #104686, #14313 ) ;
#43028=DIRECTION ( 'NONE',  ( 0.000000000000000000, 0.7071067811865466846, 0.7071067811865484609 ) ) ;
#43151=VECTOR ( 'NONE', #82773, 1000.000000000000000 ) ;
#43377=FACE_OUTER_BOUND ( 'NONE', #65455, .T. ) ;
#43416=SURFACE_STYLE_FILL_AREA ( #135441 ) ;
#43515=CYLINDRICAL_SURFACE ( 'NONE', #179855, 4.999999999999999112 ) ;
#43644=ORIENTED_EDGE ( 'NONE', *, *, #31456, .T. ) ;
#43684=CARTESIAN_POINT ( 'NONE',  ( 3.889087296526329229, 29.99999999999996092, 1.818019484660534868 ) ) ;
#44169=CARTESIAN_POINT ( 'NONE',  ( 20.96320343559668942, 21.46320343559617427, 4.646446609406719830 ) ) ;
#44239=DIRECTION ( 'NONE',  ( 0.7071067811865512365, 0.7071067811865439090, -0.000000000000000000 ) ) ;
#44361=EDGE_CURVE ( 'NONE', #144525, #30159, #35200, .T. ) ;
#44451=VECTOR ( 'NONE', #74680, 1000.000000000000000 ) ;
#44613=CARTESIAN_POINT ( 'NONE',  ( 23.46320343559666100, 18.96320343559613875, 1.110912703473986074 ) ) ;
#44650=FACE_BOUND ( 'NONE', #107983, .T. ) ;
#44839=ORIENTED_EDGE ( 'NONE', *, *, #91376, .F. ) ;
#44900=CYLINDRICAL_SURFACE ( 'NONE', #111346, 7.500000000000000000 ) ;
#45028=ORIENTED_EDGE ( 'NONE', *, *, #197329, .F. ) ;
#45082=CARTESIAN_POINT ( 'NONE',  ( -7.052343178074647945, -2.552343178074588437, 1.110912703473986074 ) ) ;
#45179=CARTESIAN_POINT ( 'NONE',  ( -2.552343178074661267, -7.052343178074616858, 8.889087296526001936 ) ) ;
#45553=( BOUNDED_CURVE ( )  B_SPLINE_CURVE ( 3, ( #192198, #101164, #69846, #132521 ),
 .UNSPECIFIED., .F., .T. ) 
 B_SPLINE_CURVE_WITH_KNOTS ( ( 4, 4 ),
 ( 1.132647296210725241, 2.115944711806982959 ),
 .UNSPECIFIED. ) 
 CURVE ( )  GEOMETRIC_REPRESENTATION_ITEM ( )  RATIONAL_B_SPLINE_CURVE ( ( 1.000000000000000000, 0.9210371567966660900, 0.9210371567966660900, 1.000000000000000000 ) ) 
 REPRESENTATION_ITEM ( '' )  );
#45637=CARTESIAN_POINT ( 'NONE',  ( -3.889087296525651105, 35.00000000000004263, 8.181980515339454030 ) ) ;
#45713=VERTEX_POINT ( 'NONE', #184434 ) ;
#45740=DIRECTION ( 'NONE',  ( -0.5000000000000002220, -0.4999999999999985012, 0.7071067811865483499 ) ) ;
#45804=ORIENTED_EDGE ( 'NONE', *, *, #35688, .T. ) ;
#46039=VERTEX_POINT ( 'NONE', #86683 ) ;
#46389=CARTESIAN_POINT ( 'NONE',  ( 6.791538853603070081, -3.181980515339468241, 1.110912703473986074 ) ) ;
#46585=CIRCLE ( 'NONE', #40085, 5.000000000000000000 ) ;
#46691=DIRECTION ( 'NONE',  ( -0.7071067811865466846, 2.468850131082262977E-15, 0.7071067811865484609 ) ) ;
#46709=ORIENTED_EDGE ( 'NONE', *, *, #152294, .F. ) ;
#46840=VECTOR ( 'NONE', #189925, 1000.000000000000000 ) ;
#46946=ORIENTED_EDGE ( 'NONE', *, *, #137445, .F. ) ;
#47105=FACE_OUTER_BOUND ( 'NONE', #22670, .T. ) ;
#47247=AXIS2_PLACEMENT_3D ( 'NONE', #26660, #9490, #118662 ) ;
#47436=DIRECTION ( 'NONE',  ( -0.7071067811865561215, -0.7071067811865389130, -0.000000000000000000 ) ) ;
#47569=LINE ( 'NONE', #173900, #156416 ) ;
#47620=DIRECTION ( 'NONE',  ( 0.7071067811865414665, -0.7071067811865536790, -0.000000000000000000 ) ) ;
#47714=ORIENTED_EDGE ( 'NONE', *, *, #168500, .F. ) ;
#47741=CARTESIAN_POINT ( 'NONE',  ( -3.660253528765646358, -6.551653823223124284, 1.589185716900144207 ) ) ;
#47748=CARTESIAN_POINT ( 'NONE',  ( 21.46320343559668231, 20.96320343559617072, 5.353553390593268624 ) ) ;
#47855=PLANE ( 'NONE',  #191436 ) ;
#48058=PLANE ( 'NONE',  #41047 ) ;
#48667=EDGE_CURVE ( 'NONE', #128792, #30636, #137115, .T. ) ;
#48939=DIRECTION ( 'NONE',  ( -1.000000000000000000, -0.000000000000000000, -0.000000000000000000 ) ) ;
#48994=VERTEX_POINT ( 'NONE', #130325 ) ;
#49117=DIRECTION ( 'NONE',  ( 0.000000000000000000, -0.8164965809277251463, 0.5773502691896268413 ) ) ;
#49436=PLANE ( 'NONE',  #51489 ) ;
#49568=CARTESIAN_POINT ( 'NONE',  ( 6.412877669190332419, 3.889087296526017479, 8.181980515339454030 ) ) ;
#49709=AXIS2_PLACEMENT_3D ( 'NONE', #158220, #126870, #144038 ) ;
#49938=ORIENTED_EDGE ( 'NONE', *, *, #112694, .F. ) ;
#49980=CARTESIAN_POINT ( 'NONE',  ( 24.49873734152912519, -24.99873734152920690, 5.353553390593271288 ) ) ;
#50035=VECTOR ( 'NONE', #65378, 1000.000000000000000 ) ;
#50048=CARTESIAN_POINT ( 'NONE',  ( -4.962140900324383708, 6.180203150055898931, 3.431593142121020623 ) ) ;
#50088=DIRECTION ( 'NONE',  ( 0.7071067811865467956, -2.468850131082262977E-15, -0.7071067811865483499 ) ) ;
#50134=AXIS2_PLACEMENT_3D ( 'NONE', #148170, #166341, #135993 ) ;
#50224=DIRECTION ( 'NONE',  ( 0.8164965809277242581, 0.000000000000000000, -0.5773502691896281735 ) ) ;
#50238=VERTEX_POINT ( 'NONE', #127109 ) ;
#50415=AXIS2_PLACEMENT_3D ( 'NONE', #184297, #105463, #154940 ) ;
#50444=CARTESIAN_POINT ( 'NONE',  ( 24.49873734152912874, -24.99873734152920690, 5.353553390593267736 ) ) ;
#50457=CARTESIAN_POINT ( 'NONE',  ( -7.500000000000001776, 1.104226503365435264, 3.188666715448012834 ) ) ;
#50513=CARTESIAN_POINT ( 'NONE',  ( -20.96320343559654020, -21.46320343559631638, 4.646446609406719830 ) ) ;
#50677=APPLICATION_CONTEXT ( 'automotive_design' ) ;
#50847=CARTESIAN_POINT ( 'NONE',  ( 2.552343178074615970, -7.052343178074640839, 1.110912703473986074 ) ) ;
#50924=LINE ( 'NONE', #35745, #85622 ) ;
#51072=PLANE ( 'NONE',  #194786 ) ;
#51096=DIRECTION ( 'NONE',  ( -0.7071067811865467956, 0.000000000000000000, -0.7071067811865483499 ) ) ;
#51432=EDGE_CURVE ( 'NONE', #133752, #6681, #159608, .T. ) ;
#51489=AXIS2_PLACEMENT_3D ( 'NONE', #32283, #108108, #186982 ) ;
#51619=CARTESIAN_POINT ( 'NONE',  ( -3.889087296526037463, -6.412877669190318208, 1.818019484660534424 ) ) ;
#51714=DIRECTION ( 'NONE',  ( -0.4999999999999978906, 0.5000000000000033307, -0.7071067811865466846 ) ) ;
#51780=DIRECTION ( 'NONE',  ( 0.7071067811865466846, -2.468850131082262977E-15, -0.7071067811865484609 ) ) ;
#51781=ORIENTED_EDGE ( 'NONE', *, *, #112155, .F. ) ;
#51867=DIRECTION ( 'NONE',  ( -0.000000000000000000, -0.000000000000000000, 1.000000000000000000 ) ) ;
#51904=VERTEX_POINT ( 'NONE', #140571 ) ;
#52031=FACE_OUTER_BOUND ( 'NONE', #19960, .T. ) ;
#52032=( BOUNDED_CURVE ( )  B_SPLINE_CURVE ( 3, ( #191239, #81053, #116391, #174088 ),
 .UNSPECIFIED., .F., .T. ) 
 B_SPLINE_CURVE_WITH_KNOTS ( ( 4, 4 ),
 ( 1.132647296210725907, 2.115944711806982959 ),
 .UNSPECIFIED. ) 
 CURVE ( )  GEOMETRIC_REPRESENTATION_ITEM ( )  RATIONAL_B_SPLINE_CURVE ( ( 1.000000000000000000, 0.9210371567966660900, 0.9210371567966660900, 1.000000000000000000 ) ) 
 REPRESENTATION_ITEM ( '' )  );
#52207=EDGE_LOOP ( 'NONE', ( #12421, #148348, #17220, #34239, #195689 ) ) ;
#52643=EDGE_CURVE ( 'NONE', #79638, #48994, #175795, .T. ) ;
#52658=CARTESIAN_POINT ( 'NONE',  ( -7.500000000000000000, 0.000000000000000000, 10.00000000000000000 ) ) ;
#52893=EDGE_LOOP ( 'NONE', ( #33146, #199013, #118504, #119376, #88322, #115775, #118596, #21394, #113655, #57111, #121428, #97638 ) ) ;
#52906=VERTEX_POINT ( 'NONE', #72727 ) ;
#53195=CARTESIAN_POINT ( 'NONE',  ( -21.46320343559624533, 20.96320343559661481, 4.646446609406720718 ) ) ;
#53222=( BOUNDED_CURVE ( )  B_SPLINE_CURVE ( 3, ( #182032, #40523, #58671, #57699 ),
 .UNSPECIFIED., .F., .F. ) 
 B_SPLINE_CURVE_WITH_KNOTS ( ( 4, 4 ),
 ( 2.008945357379066543, 2.115944711806982070 ),
 .UNSPECIFIED. ) 
 CURVE ( )  GEOMETRIC_REPRESENTATION_ITEM ( )  RATIONAL_B_SPLINE_CURVE ( ( 1.000000000000000000, 0.9990461557208837329, 0.9990461557208837329, 1.000000000000000000 ) ) 
 REPRESENTATION_ITEM ( '' )  );
#53288=VECTOR ( 'NONE', #36079, 999.9999999999998863 ) ;
#53457=CARTESIAN_POINT ( 'NONE',  ( -1.784589286804288299, -7.284589286804248331, 8.181980515339454030 ) ) ;
#53820=CARTESIAN_POINT ( 'NONE',  ( -7.052343178074647945, -2.552343178074588437, 1.110912703473986074 ) ) ;
#53952=CARTESIAN_POINT ( 'NONE',  ( 6.677994727576217926, 3.424326230466338661, 8.646741581399133736 ) ) ;
#53965=DIRECTION ( 'NONE',  ( -0.7071067811865463515, 0.7071067811865487940, -0.000000000000000000 ) ) ;
#54030=ORIENTED_EDGE ( 'NONE', *, *, #48667, .T. ) ;
#54280=( GEOMETRIC_REPRESENTATION_CONTEXT ( 3 ) GLOBAL_UNCERTAINTY_ASSIGNED_CONTEXT ( ( #191473 ) ) GLOBAL_UNIT_ASSIGNED_CONTEXT ( ( #167752, #59558, #89912 ) ) REPRESENTATION_CONTEXT ( 'NONE', 'WORKASPACE' ) );
#54394=CARTESIAN_POINT ( 'NONE',  ( -24.49873734152895111, 24.99873734152937743, 5.353553390593269512 ) ) ;
#54491=DIRECTION ( 'NONE',  ( 0.4999999999999967248, -0.5000000000000019984, -0.7071067811865484609 ) ) ;
#54526=ORIENTED_EDGE ( 'NONE', *, *, #139056, .F. ) ;
#54842=CARTESIAN_POINT ( 'NONE',  ( 7.284589286804292740, 1.784589286804177277, 1.818019484660534424 ) ) ;
#54851=DIRECTION ( 'NONE',  ( 0.4999999999999932276, -0.5000000000000055511, 0.7071067811865484609 ) ) ;
#55065=CARTESIAN_POINT ( 'NONE',  ( 3.181980515339539295, 6.791538853603031889, 1.110912703473986074 ) ) ;
#55236=( BOUNDED_CURVE ( )  B_SPLINE_CURVE ( 3, ( #20858, #36023, #188739, #160375 ),
 .UNSPECIFIED., .F., .F. ) 
 B_SPLINE_CURVE_WITH_KNOTS ( ( 4, 4 ),
 ( 1.132647296210725907, 2.115944711806982514 ),
 .UNSPECIFIED. ) 
 CURVE ( )  GEOMETRIC_REPRESENTATION_ITEM ( )  RATIONAL_B_SPLINE_CURVE ( ( 1.000000000000000000, 0.9210371567966662010, 0.9210371567966662010, 1.000000000000000000 ) ) 
 REPRESENTATION_ITEM ( '' )  );
#55457=DIRECTION ( 'NONE',  ( 0.7071067811865483499, 0.000000000000000000, -0.7071067811865465735 ) ) ;
#55488=DIRECTION ( 'NONE',  ( -0.7071067811865483499, 0.000000000000000000, 0.7071067811865465735 ) ) ;
#55576=DIRECTION ( 'NONE',  ( 3.491481338843133750E-15, 1.000000000000000000, -0.000000000000000000 ) ) ;
#55714=CARTESIAN_POINT ( 'NONE',  ( 7.128481858827110607, -2.709097808555395392, 2.998008972631150737 ) ) ;
#55984=AXIS2_PLACEMENT_3D ( 'NONE', #42291, #14925, #182789 ) ;
#56096=VERTEX_POINT ( 'NONE', #53457 ) ;
#56337=FACE_OUTER_BOUND ( 'NONE', #68324, .T. ) ;
#56557=CARTESIAN_POINT ( 'NONE',  ( 7.284589286804261654, -1.784589286804270980, 8.181980515339454030 ) ) ;
#56646=LINE ( 'NONE', #86970, #15152 ) ;
#56725=EDGE_CURVE ( 'NONE', #26126, #103419, #172755, .T. ) ;
#56848=EDGE_CURVE ( 'NONE', #191847, #122157, #82372, .T. ) ;
#56862=CARTESIAN_POINT ( 'NONE',  ( -7.284589286804265207, -1.784589286804211916, 1.818019484660534424 ) ) ;
#56871=DIRECTION ( 'NONE',  ( 0.7071067811865467956, -7.406550393246786959E-15, 0.7071067811865483499 ) ) ;
#57111=ORIENTED_EDGE ( 'NONE', *, *, #141068, .F. ) ;
#57355=EDGE_CURVE ( 'NONE', #4626, #37612, #180825, .T. ) ;
#57395=ORIENTED_EDGE ( 'NONE', *, *, #35688, .F. ) ;
#57516=CARTESIAN_POINT ( 'NONE',  ( 26.99873734152913229, -22.49873734152921045, 8.889087296526001936 ) ) ;
#57699=CARTESIAN_POINT ( 'NONE',  ( 7.284589286804292740, 1.784589286804177277, 1.818019484660534424 ) ) ;
#57715=DIRECTION ( 'NONE',  ( 1.000000000000000000, 0.000000000000000000, 0.000000000000000000 ) ) ;
#58091=CARTESIAN_POINT ( 'NONE',  ( -3.889087296525950421, 6.412877669190374164, 8.181980515339454030 ) ) ;
#58196=PLANE ( 'NONE',  #29121 ) ;
#58262=DIRECTION ( 'NONE',  ( 0.000000000000000000, -0.7071067811865483499, -0.7071067811865465735 ) ) ;
#58377=ORIENTED_EDGE ( 'NONE', *, *, #114876, .T. ) ;
#58459=EDGE_CURVE ( 'NONE', #199067, #191847, #65400, .T. ) ;
#58517=VERTEX_POINT ( 'NONE', #11743 ) ;
#58671=CARTESIAN_POINT ( 'NONE',  ( 7.220908937440039033, 2.044528755335607073, 1.589185716900142209 ) ) ;
#58678=VERTEX_POINT ( 'NONE', #74392 ) ;
#58921=DIRECTION ( 'NONE',  ( 0.000000000000000000, -0.8164965809277253683, 0.5773502691896268413 ) ) ;
#59466=FACE_OUTER_BOUND ( 'NONE', #134762, .T. ) ;
#59558=( NAMED_UNIT ( * ) PLANE_ANGLE_UNIT ( ) SI_UNIT ( $, .RADIAN. ) );
#59561=DIRECTION ( 'NONE',  ( 0.7071067811865467956, -2.468850131082262977E-15, -0.7071067811865483499 ) ) ;
#59605=ADVANCED_FACE ( 'NONE', ( #151000 ), #164172, .T. ) ;
#59666=ORIENTED_EDGE ( 'NONE', *, *, #86587, .T. ) ;
#59682=VECTOR ( 'NONE', #71017, 1000.000000000000000 ) ;
#59712=AXIS2_PLACEMENT_3D ( 'NONE', #161996, #23492, #75707 ) ;
#59729=SURFACE_STYLE_FILL_AREA ( #74910 ) ;
#59755=CARTESIAN_POINT ( 'NONE',  ( 0.000000000000000000, 0.000000000000000000, -20.00000000000000000 ) ) ;
#59821=CARTESIAN_POINT ( 'NONE',  ( -4.962140900324464532, -6.180203150055834094, 6.568406857878973604 ) ) ;
#59872=VECTOR ( 'NONE', #121593, 1000.000000000000000 ) ;
#59967=FACE_OUTER_BOUND ( 'NONE', #132662, .T. ) ;
#60033=CARTESIAN_POINT ( 'NONE',  ( 35.00000000000000000, -0.3535533905932703447, 5.353553390593268624 ) ) ;
#60638=DIRECTION ( 'NONE',  ( -0.000000000000000000, 0.7071067811865467956, 0.7071067811865483499 ) ) ;
#60651=VERTEX_POINT ( 'NONE', #169108 ) ;
#60688=EDGE_LOOP ( 'NONE', ( #169373, #166940, #97265, #145634 ) ) ;
#60742=DIRECTION ( 'NONE',  ( -1.000000000000000000, 0.000000000000000000, 0.000000000000000000 ) ) ;
#60779=ORIENTED_EDGE ( 'NONE', *, *, #40219, .F. ) ;
#60792=DIRECTION ( 'NONE',  ( -1.047444401652940164E-14, -1.000000000000000000, -0.000000000000000000 ) ) ;
#60900=VECTOR ( 'NONE', #5513, 1000.000000000000000 ) ;
#60906=DIRECTION ( 'NONE',  ( -0.7071067811865463515, 0.7071067811865487940, -0.000000000000000000 ) ) ;
#60988=AXIS2_PLACEMENT_3D ( 'NONE', #150721, #85022, #57715 ) ;
#61062=LINE ( 'NONE', #138898, #72954 ) ;
#61151=DIRECTION ( 'NONE',  ( -0.000000000000000000, -0.000000000000000000, 1.000000000000000000 ) ) ;
#61198=ORIENTED_EDGE ( 'NONE', *, *, #183156, .F. ) ;
#61406=ORIENTED_EDGE ( 'NONE', *, *, #56848, .F. ) ;
#61612=DIRECTION ( 'NONE',  ( 0.000000000000000000, -0.8164965809277251463, 0.5773502691896268413 ) ) ;
#61796=DIRECTION ( 'NONE',  ( 0.5000000000000002220, 0.4999999999999985012, -0.7071067811865483499 ) ) ;
#62098=ORIENTED_EDGE ( 'NONE', *, *, #149135, .F. ) ;
#62204=FACE_OUTER_BOUND ( 'NONE', #96660, .T. ) ;
#62725=AXIS2_PLACEMENT_3D ( 'NONE', #59755, #11295, #184106 ) ;
#62793=CARTESIAN_POINT ( 'NONE',  ( 22.49873734152911453, -26.99873734152921045, 1.110912703473986074 ) ) ;
#62912=ORIENTED_EDGE ( 'NONE', *, *, #89293, .F. ) ;
#62966=ORIENTED_EDGE ( 'NONE', *, *, #123454, .F. ) ;
#63046=DIRECTION ( 'NONE',  ( 0.7071067811865466846, -7.406550393246786959E-15, 0.7071067811865484609 ) ) ;
#63277=PLANE ( 'NONE',  #114653 ) ;
#63719=ORIENTED_EDGE ( 'NONE', *, *, #36310, .F. ) ;
#63777=CARTESIAN_POINT ( 'NONE',  ( 7.284589286804292740, 1.784589286804177277, 1.818019484660534424 ) ) ;
#63870=DIRECTION ( 'NONE',  ( 0.8164965809277243691, 0.000000000000000000, -0.5773502691896280625 ) ) ;
#63977=ADVANCED_FACE ( 'NONE', ( #33872 ), #48058, .T. ) ;
#64097=ORIENTED_EDGE ( 'NONE', *, *, #51432, .T. ) ;
#64133=LINE ( 'NONE', #156137, #150848 ) ;
#64212=DIRECTION ( 'NONE',  ( 0.4999999999999945599, -0.5000000000000066613, -0.7071067811865467956 ) ) ;
#64222=CARTESIAN_POINT ( 'NONE',  ( -2.552343178074577779, 7.052343178074668373, 1.110912703473986074 ) ) ;
#64316=CARTESIAN_POINT ( 'NONE',  ( -2.300691058039471937, -7.143419655154863435, 8.646741581399126630 ) ) ;
#64369=DIRECTION ( 'NONE',  ( 0.000000000000000000, -0.8164965809277253683, 0.5773502691896268413 ) ) ;
#64388=PLANE ( 'NONE',  #167042 ) ;
#64459=AXIS2_PLACEMENT_3D ( 'NONE', #107520, #152060, #73253 ) ;
#64586=CARTESIAN_POINT ( 'NONE',  ( 27.49873734152943427, 21.99873734152882676, 1.818019484660534424 ) ) ;
#64613=ADVANCED_FACE ( 'NONE', ( #62204 ), #108719, .T. ) ;
#64638=ADVANCED_FACE ( 'NONE', ( #93541 ), #140039, .T. ) ;
#64689=VERTEX_POINT ( 'NONE', #5503 ) ;
#64857=ORIENTED_EDGE ( 'NONE', *, *, #157461, .F. ) ;
#64996=DIRECTION ( 'NONE',  ( -1.000000000000000000, 0.000000000000000000, 0.000000000000000000 ) ) ;
#65048=CYLINDRICAL_SURFACE ( 'NONE', #149803, 4.500000000000000000 ) ;
#65087=CARTESIAN_POINT ( 'NONE',  ( 3.181980515339539295, 6.791538853603031889, 1.110912703473986074 ) ) ;
#65227=FACE_OUTER_BOUND ( 'NONE', #167174, .T. ) ;
#65378=DIRECTION ( 'NONE',  ( -1.000000000000000000, -0.000000000000000000, -0.000000000000000000 ) ) ;
#65386=ORIENTED_EDGE ( 'NONE', *, *, #162333, .T. ) ;
#65400=LINE ( 'NONE', #69388, #72761 ) ;
#65432=EDGE_LOOP ( 'NONE', ( #157295, #40743, #124777, #27375 ) ) ;
#65455=EDGE_LOOP ( 'NONE', ( #127830, #20188, #139134, #116669 ) ) ;
#65531=CARTESIAN_POINT ( 'NONE',  ( -0.3535533905933929688, -35.00000000000000000, 5.353553390593268624 ) ) ;
#65912=( GEOMETRIC_REPRESENTATION_CONTEXT ( 3 ) GLOBAL_UNCERTAINTY_ASSIGNED_CONTEXT ( ( #37796 ) ) GLOBAL_UNIT_ASSIGNED_CONTEXT ( ( #190273, #144751, #100247 ) ) REPRESENTATION_CONTEXT ( 'NONE', 'WORKASPACE' ) );
#66079=DIRECTION ( 'NONE',  ( 0.000000000000000000, -0.7071067811865483499, -0.7071067811865466846 ) ) ;
#66130=CARTESIAN_POINT ( 'NONE',  ( -7.143419655154851888, 2.300691058039502135, 8.646741581399137289 ) ) ;
#66201=DIRECTION ( 'NONE',  ( 0.000000000000000000, -0.8164965809277252573, 0.5773502691896267303 ) ) ;
#66237=FACE_OUTER_BOUND ( 'NONE', #177929, .T. ) ;
#66629=CARTESIAN_POINT ( 'NONE',  ( 0.000000000000000000, 0.000000000000000000, 0.000000000000000000 ) ) ;
#66660=DIRECTION ( 'NONE',  ( 2.081668171172168513E-15, -0.8164965809277244801, 0.5773502691896279515 ) ) ;
#66710=DIRECTION ( 'NONE',  ( 0.7071067811865483499, 2.636779683484746468E-14, -0.7071067811865465735 ) ) ;
#66728=LINE ( 'NONE', #68717, #172681 ) ;
#66990=CARTESIAN_POINT ( 'NONE',  ( 3.889087296526082316, 6.412877669190294228, 1.818019484660534424 ) ) ;
#67115=CARTESIAN_POINT ( 'NONE',  ( 3.181980515339834614, 34.99999999999997158, 1.110912703473986074 ) ) ;
#67128=CARTESIAN_POINT ( 'NONE',  ( 26.99873734152913229, -22.49873734152921045, 8.889087296526001936 ) ) ;
#67252=DIRECTION ( 'NONE',  ( 0.7071067811865466846, -2.468850131082262977E-15, -0.7071067811865484609 ) ) ;
#67374=EDGE_CURVE ( 'NONE', #27352, #133752, #185997, .T. ) ;
#67610=ORIENTED_EDGE ( 'NONE', *, *, #52643, .T. ) ;
#67630=DIRECTION ( 'NONE',  ( 0.7071067811865483499, 0.000000000000000000, -0.7071067811865466846 ) ) ;
#67879=CARTESIAN_POINT ( 'NONE',  ( 7.500000000000000888, -1.380023386739103852, 4.327083394447440057 ) ) ;
#68066=EDGE_LOOP ( 'NONE', ( #113417, #80674, #58377, #183854 ) ) ;
#68097=ORIENTED_EDGE ( 'NONE', *, *, #73850, .F. ) ;
#68207=( BOUNDED_CURVE ( )  B_SPLINE_CURVE ( 3, ( #22083, #19107, #3913, #83734 ),
 .UNSPECIFIED., .F., .F. ) 
 B_SPLINE_CURVE_WITH_KNOTS ( ( 4, 4 ),
 ( 1.025647941782810824, 1.570796326794896558 ),
 .UNSPECIFIED. ) 
 CURVE ( )  GEOMETRIC_REPRESENTATION_ITEM ( )  RATIONAL_B_SPLINE_CURVE ( ( 1.000000000000000000, 0.9753873905749756990, 0.9753873905749756990, 1.000000000000000000 ) ) 
 REPRESENTATION_ITEM ( '' )  );
#68324=EDGE_LOOP ( 'NONE', ( #18598, #198466, #173582, #130520 ) ) ;
#68449=ORIENTED_EDGE ( 'NONE', *, *, #41619, .T. ) ;
#68552=DIRECTION ( 'NONE',  ( -0.000000000000000000, -0.000000000000000000, -1.000000000000000000 ) ) ;
#68569=CARTESIAN_POINT ( 'NONE',  ( 2.552343178074615970, -7.052343178074640839, 1.110912703473986074 ) ) ;
#68717=CARTESIAN_POINT ( 'NONE',  ( -35.00000000000000000, -3.181980515339470905, 8.889087296526001936 ) ) ;
#68944=DIRECTION ( 'NONE',  ( 0.000000000000000000, -0.7071067811865483499, -0.7071067811865465735 ) ) ;
#69111=CARTESIAN_POINT ( 'NONE',  ( 6.412877669190332419, 3.889087296526017479, 8.181980515339454030 ) ) ;
#69253=DIRECTION ( 'NONE',  ( 0.7071067811865483499, -7.406550393246807469E-15, -0.7071067811865467956 ) ) ;
#69380=CIRCLE ( 'NONE', #153380, 5.000000000000000888 ) ;
#69388=CARTESIAN_POINT ( 'NONE',  ( -3.889087296525703508, 30.00000000000004263, 8.181980515339454030 ) ) ;
#69761=DIRECTION ( 'NONE',  ( 0.7071067811865414665, -0.7071067811865536790, -0.000000000000000000 ) ) ;
#69846=CARTESIAN_POINT ( 'NONE',  ( 6.674792076160520615, -4.273745901508142708, 5.990689250852172520 ) ) ;
#69902=EDGE_LOOP ( 'NONE', ( #32299, #24832, #114292, #142539 ) ) ;
#69929=EDGE_CURVE ( 'NONE', #157949, #89709, #55236, .T. ) ;
#70007=ADVANCED_FACE ( 'NONE', ( #110881 ), #64388, .T. ) ;
#70148=LINE ( 'NONE', #195510, #21384 ) ;
#70200=ORIENTED_EDGE ( 'NONE', *, *, #51432, .F. ) ;
#70454=ORIENTED_EDGE ( 'NONE', *, *, #55, .T. ) ;
#70728=DIRECTION ( 'NONE',  ( -0.5000000000000002220, -0.4999999999999985567, 0.7071067811865484609 ) ) ;
#70794=CARTESIAN_POINT ( 'NONE',  ( 0.8613000766924048257, -7.878827036337491485, 6.568406857878970939 ) ) ;
#70918=ORIENTED_EDGE ( 'NONE', *, *, #141068, .T. ) ;
#71017=DIRECTION ( 'NONE',  ( 0.000000000000000000, 0.7071067811865467956, -0.7071067811865483499 ) ) ;
#71166=ORIENTED_EDGE ( 'NONE', *, *, #18906, .T. ) ;
#71353=CARTESIAN_POINT ( 'NONE',  ( 7.500000000000000000, 9.184850993605147944E-16, 10.00000000000000000 ) ) ;
#71612=ORIENTED_EDGE ( 'NONE', *, *, #183693, .T. ) ;
#71629=CARTESIAN_POINT ( 'NONE',  ( -1.784589286804201480, 7.284589286804282970, 1.818019484660534424 ) ) ;
#71744=LINE ( 'NONE', #7056, #181795 ) ;
#71897=ORIENTED_EDGE ( 'NONE', *, *, #37374, .F. ) ;
#72094=EDGE_CURVE ( 'NONE', #46039, #4246, #111922, .T. ) ;
#72124=DIRECTION ( 'NONE',  ( 0.4999999999999933387, -0.5000000000000055511, 0.7071067811865484609 ) ) ;
#72170=ORIENTED_EDGE ( 'NONE', *, *, #112694, .T. ) ;
#72193=ADVANCED_FACE ( 'NONE', ( #159598 ), #20100, .T. ) ;
#72309=AXIS2_PLACEMENT_3D ( 'NONE', #129302, #173854, #95994 ) ;
#72517=CYLINDRICAL_SURFACE ( 'NONE', #134066, 5.000000000000000000 ) ;
#72574=AXIS2_PLACEMENT_3D ( 'NONE', #13272, #89108, #12294 ) ;
#72698=CIRCLE ( 'NONE', #150207, 4.999999999999998224 ) ;
#72727=CARTESIAN_POINT ( 'NONE',  ( 2.552343178074723884, 7.052343178074616858, 8.889087296526001936 ) ) ;
#72739=VECTOR ( 'NONE', #92475, 999.9999999999998863 ) ;
#72761=VECTOR ( 'NONE', #127061, 1000.000000000000000 ) ;
#72888=AXIS2_PLACEMENT_3D ( 'NONE', #20134, #143466, #67630 ) ;
#72939=( NAMED_UNIT ( * ) SI_UNIT ( $, .STERADIAN. ) SOLID_ANGLE_UNIT ( ) );
#72954=VECTOR ( 'NONE', #169236, 1000.000000000000000 ) ;
#73001=CARTESIAN_POINT ( 'NONE',  ( -20.96320343559654020, -25.54568634023494411, 7.533197955354854258 ) ) ;
#73125=ORIENTED_EDGE ( 'NONE', *, *, #168721, .F. ) ;
#73182=ORIENTED_EDGE ( 'NONE', *, *, #114876, .F. ) ;
#73245=AXIS2_PLACEMENT_3D ( 'NONE', #1528, #64212, #82332 ) ;
#73250=CARTESIAN_POINT ( 'NONE',  ( 6.412877669190335972, -3.889087296526014814, 1.818019484660534424 ) ) ;
#73253=DIRECTION ( 'NONE',  ( -1.000000000000000000, 0.000000000000000000, 0.000000000000000000 ) ) ;
#73359=VECTOR ( 'NONE', #112103, 1000.000000000000000 ) ;
#73511=AXIS2_PLACEMENT_3D ( 'NONE', #196479, #14408, #119620 ) ;
#73604=ADVANCED_FACE ( 'NONE', ( #91221 ), #152912, .T. ) ;
#73850=EDGE_CURVE ( 'NONE', #33153, #42657, #12454, .T. ) ;
#73924=( BOUNDED_CURVE ( )  B_SPLINE_CURVE ( 3, ( #22425, #84075, #5238, #7236 ),
 .UNSPECIFIED., .F., .F. ) 
 B_SPLINE_CURVE_WITH_KNOTS ( ( 4, 4 ),
 ( 5.150538010968860547, 5.257537365396776075 ),
 .UNSPECIFIED. ) 
 CURVE ( )  GEOMETRIC_REPRESENTATION_ITEM ( )  RATIONAL_B_SPLINE_CURVE ( ( 1.000000000000000000, 0.9990461557208837329, 0.9990461557208837329, 1.000000000000000000 ) ) 
 REPRESENTATION_ITEM ( '' )  );
#73932=SHAPE_REPRESENTATION_RELATIONSHIP ( 'NONE' , 'NONE' ,  #8335, #117169 ) ;
#74086=ORIENTED_EDGE ( 'NONE', *, *, #156994, .F. ) ;
#74204=CARTESIAN_POINT ( 'NONE',  ( -6.412877669190332419, -3.889087296526017479, 8.181980515339454030 ) ) ;
#74277=DIRECTION ( 'NONE',  ( 0.000000000000000000, 0.000000000000000000, 1.000000000000000000 ) ) ;
#74392=CARTESIAN_POINT ( 'NONE',  ( -24.99873734152929217, -24.49873734152903282, 5.353553390593269512 ) ) ;
#74443=DIRECTION ( 'NONE',  ( 1.000000000000000000, -0.000000000000000000, -0.000000000000000000 ) ) ;
#74465=CIRCLE ( 'NONE', #96937, 5.000000000000000000 ) ;
#74680=DIRECTION ( 'NONE',  ( -0.000000000000000000, -0.000000000000000000, -1.000000000000000000 ) ) ;
#74703=DIRECTION ( 'NONE',  ( 0.4999999999999966693, -0.5000000000000019984, -0.7071067811865483499 ) ) ;
#74910=FILL_AREA_STYLE ('',( #41598 ) ) ;
#74983=FACE_BOUND ( 'NONE', #27439, .T. ) ;
#75231=CARTESIAN_POINT ( 'NONE',  ( 7.500000000000000000, 9.184850993605147944E-16, 0.000000000000000000 ) ) ;
#75343=VERTEX_POINT ( 'NONE', #104208 ) ;
#75551=CARTESIAN_POINT ( 'NONE',  ( -6.412877669190335972, 3.889087296526014814, 1.818019484660534424 ) ) ;
#75603=PLANE ( 'NONE',  #173649 ) ;
#75707=DIRECTION ( 'NONE',  ( 0.8164965809277243691, 0.000000000000000000, -0.5773502691896280625 ) ) ;
#75717=AXIS2_PLACEMENT_3D ( 'NONE', #162957, #86113, #147804 ) ;
#75724=PRESENTATION_STYLE_ASSIGNMENT (( #124212 ) ) ;
#75757=EDGE_LOOP ( 'NONE', ( #191246, #14812, #101514, #22192 ) ) ;
#75898=ORIENTED_EDGE ( 'NONE', *, *, #44361, .F. ) ;
#76338=AXIS2_PLACEMENT_3D ( 'NONE', #161208, #111716, #66201 ) ;
#76400=CARTESIAN_POINT ( 'NONE',  ( -7.284589286804265207, -1.784589286804211916, 1.818019484660534424 ) ) ;
#76583=ORIENTED_EDGE ( 'NONE', *, *, #168500, .T. ) ;
#76674=DIRECTION ( 'NONE',  ( 0.000000000000000000, -0.7071067811865466846, 0.7071067811865484609 ) ) ;
#76836=CARTESIAN_POINT ( 'NONE',  ( -7.500000000000000000, 0.000000000000000000, 4.292893218813445877 ) ) ;
#77150=ORIENTED_EDGE ( 'NONE', *, *, #172493, .F. ) ;
#77182=CARTESIAN_POINT ( 'NONE',  ( 35.00000000000000000, 3.181980515339470905, 8.889087296526001936 ) ) ;
#77367=ORIENTED_EDGE ( 'NONE', *, *, #4454, .F. ) ;
#77575=ORIENTED_EDGE ( 'NONE', *, *, #173518, .F. ) ;
#77655=CARTESIAN_POINT ( 'NONE',  ( 2.300691058039529224, 7.143419655154843007, 8.646741581399139065 ) ) ;
#77715=SURFACE_SIDE_STYLE ('',( #43416 ) ) ;
#77946=FACE_OUTER_BOUND ( 'NONE', #127929, .T. ) ;
#77964=CARTESIAN_POINT ( 'NONE',  ( -2.552343178074661267, -7.052343178074616858, 8.889087296526001936 ) ) ;
#78005=DIRECTION ( 'NONE',  ( 0.7071067811865485719, 0.000000000000000000, 0.7071067811865465735 ) ) ;
#78169=LINE ( 'NONE', #60033, #165770 ) ;
#78497=ORIENTED_EDGE ( 'NONE', *, *, #36811, .T. ) ;
#78559=ADVANCED_FACE ( 'NONE', ( #33093 ), #75603, .T. ) ;
#78641=CARTESIAN_POINT ( 'NONE',  ( 0.000000000000000000, 0.000000000000000000, 0.000000000000000000 ) ) ;
#78642=ORIENTED_EDGE ( 'NONE', *, *, #110020, .F. ) ;
#78871=CIRCLE ( 'NONE', #98331, 5.000000000000000000 ) ;
#79023=FACE_OUTER_BOUND ( 'NONE', #65432, .T. ) ;
#79223=MANIFOLD_SOLID_BREP ( 'Boss-Extrude2', #195120 ) ;
#79512=AXIS2_PLACEMENT_3D ( 'NONE', #155808, #61796, #125481 ) ;
#79638=VERTEX_POINT ( 'NONE', #144353 ) ;
#80006=CARTESIAN_POINT ( 'NONE',  ( -6.677994727576218814, 3.424326230466335996, 1.353258418600855606 ) ) ;
#80057=DIRECTION ( 'NONE',  ( 0.4999999999999933387, -0.5000000000000055511, 0.7071067811865484609 ) ) ;
#80087=VERTEX_POINT ( 'NONE', #97829 ) ;
#80338=ORIENTED_EDGE ( 'NONE', *, *, #13111, .T. ) ;
#80542=CARTESIAN_POINT ( 'NONE',  ( 35.00000000000000000, 3.181980515339470905, 8.889087296526001936 ) ) ;
#80548=EDGE_LOOP ( 'NONE', ( #73125, #110031, #139516, #43644, #105823 ) ) ;
#80674=ORIENTED_EDGE ( 'NONE', *, *, #120835, .T. ) ;
#80759=PLANE ( 'NONE',  #144315 ) ;
#80884=DIRECTION ( 'NONE',  ( 0.000000000000000000, 0.7071067811865466846, 0.7071067811865484609 ) ) ;
#80957=DIRECTION ( 'NONE',  ( 0.7071067811865483499, 0.000000000000000000, 0.7071067811865465735 ) ) ;
#80990=CARTESIAN_POINT ( 'NONE',  ( -6.791538853603066528, 3.181980515339468241, 1.110912703473986074 ) ) ;
#81053=CARTESIAN_POINT ( 'NONE',  ( -0.8613000766924595597, -7.878827036337484380, 3.431593142121016626 ) ) ;
#81477=VERTEX_POINT ( 'NONE', #1785 ) ;
#81982=ORIENTED_EDGE ( 'NONE', *, *, #2501, .F. ) ;
#82054=AXIS2_PLACEMENT_3D ( 'NONE', #82060, #99242, #83075 ) ;
#82060=CARTESIAN_POINT ( 'NONE',  ( 0.000000000000000000, 0.000000000000000000, 0.000000000000000000 ) ) ;
#82328=AXIS2_PLACEMENT_3D ( 'NONE', #53195, #22871, #84518 ) ;
#82332=DIRECTION ( 'NONE',  ( 0.000000000000000000, 0.8164965809277221487, -0.5773502691896313932 ) ) ;
#82372=CIRCLE ( 'NONE', #40412, 5.000000000000000888 ) ;
#82470=CIRCLE ( 'NONE', #198707, 5.000000000000000888 ) ;
#82597=PRODUCT_CONTEXT ( 'NONE', #161685, 'mechanical' ) ;
#82773=DIRECTION ( 'NONE',  ( 3.491481338843133750E-15, 1.000000000000000000, -0.000000000000000000 ) ) ;
#82807=CARTESIAN_POINT ( 'NONE',  ( 6.791538853603062975, 3.181980515339470905, 8.889087296526001936 ) ) ;
#82972=VECTOR ( 'NONE', #162351, 1000.000000000000000 ) ;
#83075=DIRECTION ( 'NONE',  ( 1.000000000000000000, 0.000000000000000000, 0.000000000000000000 ) ) ;
#83148=CARTESIAN_POINT ( 'NONE',  ( -20.96320343559654020, -21.46320343559631638, 4.646446609406719830 ) ) ;
#83467=ORIENTED_EDGE ( 'NONE', *, *, #139917, .F. ) ;
#83496=DIRECTION ( 'NONE',  ( 0.000000000000000000, -0.7071067811865485719, 0.7071067811865465735 ) ) ;
#83516=DIRECTION ( 'NONE',  ( 0.5000000000000037748, 0.4999999999999950040, 0.7071067811865483499 ) ) ;
#83557=( BOUNDED_CURVE ( )  B_SPLINE_CURVE ( 3, ( #99442, #53952, #131792, #69111 ),
 .UNSPECIFIED., .F., .T. ) 
 B_SPLINE_CURVE_WITH_KNOTS ( ( 4, 4 ),
 ( 5.150538010968860547, 5.257537365396776075 ),
 .UNSPECIFIED. ) 
 CURVE ( )  GEOMETRIC_REPRESENTATION_ITEM ( )  RATIONAL_B_SPLINE_CURVE ( ( 1.000000000000000000, 0.9990461557208837329, 0.9990461557208837329, 1.000000000000000000 ) ) 
 REPRESENTATION_ITEM ( '' )  );
#83713=CARTESIAN_POINT ( 'NONE',  ( -7.500000000000000000, 0.000000000000000000, 10.00000000000000000 ) ) ;
#83734=CARTESIAN_POINT ( 'NONE',  ( -7.500000000000000000, 0.000000000000000000, 5.707106781186540800 ) ) ;
#83857=CARTESIAN_POINT ( 'NONE',  ( 25.04568634023502582, -21.46320343559646560, 8.240304736541396835 ) ) ;
#83920=( BOUNDED_CURVE ( )  B_SPLINE_CURVE ( 3, ( #50847, #113490, #5316, #35666 ),
 .UNSPECIFIED., .F., .T. ) 
 B_SPLINE_CURVE_WITH_KNOTS ( ( 4, 4 ),
 ( 2.008945357379067875, 2.115944711806982070 ),
 .UNSPECIFIED. ) 
 CURVE ( )  GEOMETRIC_REPRESENTATION_ITEM ( )  RATIONAL_B_SPLINE_CURVE ( ( 1.000000000000000000, 0.9990461557208837329, 0.9990461557208837329, 1.000000000000000000 ) ) 
 REPRESENTATION_ITEM ( '' )  );
#84075=CARTESIAN_POINT ( 'NONE',  ( 3.424326230466315568, -6.677994727576229472, 8.646741581399133736 ) ) ;
#84223=ORIENTED_EDGE ( 'NONE', *, *, #150915, .T. ) ;
#84353=DIRECTION ( 'NONE',  ( 0.4999999999999978906, -0.5000000000000033307, 0.7071067811865466846 ) ) ;
#84463=VERTEX_POINT ( 'NONE', #111946 ) ;
#84518=DIRECTION ( 'NONE',  ( 0.8164965809277243691, 0.000000000000000000, -0.5773502691896280625 ) ) ;
#84590=CARTESIAN_POINT ( 'NONE',  ( 30.00000000000000355, 3.889087296526017479, 8.181980515339454030 ) ) ;
#84701=ORIENTED_EDGE ( 'NONE', *, *, #90984, .F. ) ;
#84709=LINE ( 'NONE', #143389, #46840 ) ;
#84796=CARTESIAN_POINT ( 'NONE',  ( -4.500000000000000000, 5.510910596163088569E-16, -20.00000000000000000 ) ) ;
#84916=CARTESIAN_POINT ( 'NONE',  ( 7.284589286804261654, -1.784589286804270980, 8.181980515339454030 ) ) ;
#85022=DIRECTION ( 'NONE',  ( 0.000000000000000000, 0.000000000000000000, 1.000000000000000000 ) ) ;
#85047=VERTEX_POINT ( 'NONE', #158445 ) ;
#85282=VECTOR ( 'NONE', #96853, 1000.000000000000000 ) ;
#85440=ADVANCED_FACE ( 'NONE', ( #116929 ), #193792, .T. ) ;
#85507=FACE_OUTER_BOUND ( 'NONE', #175109, .T. ) ;
#85589=DIRECTION ( 'NONE',  ( 0.000000000000000000, -0.7071067811865466846, 0.7071067811865484609 ) ) ;
#85622=VECTOR ( 'NONE', #88236, 999.9999999999998863 ) ;
#85800=VERTEX_POINT ( 'NONE', #89590 ) ;
#85884=CARTESIAN_POINT ( 'NONE',  ( 23.96320343559640165, -18.46320343559646560, 8.181980515339454030 ) ) ;
#86113=DIRECTION ( 'NONE',  ( -0.4999999999999945599, 0.5000000000000066613, 0.7071067811865467956 ) ) ;
#86167=AXIS2_PLACEMENT_3D ( 'NONE', #116846, #23852, #145175 ) ;
#86241=VERTEX_POINT ( 'NONE', #16726 ) ;
#86511=EDGE_CURVE ( 'NONE', #85800, #199879, #153261, .T. ) ;
#86543=ORIENTED_EDGE ( 'NONE', *, *, #157461, .T. ) ;
#86587=EDGE_CURVE ( 'NONE', #17186, #166399, #148103, .T. ) ;
#86683=CARTESIAN_POINT ( 'NONE',  ( -6.791538853603066528, 3.181980515339468241, 1.110912703473986074 ) ) ;
#86775=ORIENTED_EDGE ( 'NONE', *, *, #172493, .T. ) ;
#86800=CARTESIAN_POINT ( 'NONE',  ( -35.00000000000000000, 3.889087296526014814, 1.818019484660534424 ) ) ;
#86872=CARTESIAN_POINT ( 'NONE',  ( 21.46320343559639454, -20.96320343559646915, 4.646446609406721606 ) ) ;
#86970=CARTESIAN_POINT ( 'NONE',  ( -30.00000000000000355, 3.889087296526015258, 1.818019484660534646 ) ) ;
#87117=EDGE_CURVE ( 'NONE', #26126, #36918, #173940, .T. ) ;
#87134=EDGE_CURVE ( 'NONE', #13627, #36918, #173397, .T. ) ;
#87189=DIRECTION ( 'NONE',  ( 0.000000000000000000, -0.8164965809277233699, -0.5773502691896295058 ) ) ;
#87267=AXIS2_PLACEMENT_3D ( 'NONE', #37783, #177321, #115632 ) ;
#87279=CARTESIAN_POINT ( 'NONE',  ( -23.46320343559652954, -18.96320343559629507, 1.110912703473986074 ) ) ;
#87361=VECTOR ( 'NONE', #42031, 1000.000000000000114 ) ;
#87398=FACE_OUTER_BOUND ( 'NONE', #97759, .T. ) ;
#87570=ORIENTED_EDGE ( 'NONE', *, *, #179632, .F. ) ;
#87603=CARTESIAN_POINT ( 'NONE',  ( -35.00000000000000000, 3.181980515339468241, 1.110912703473986074 ) ) ;
#87873=PLANE ( 'NONE',  #121146 ) ;
#87874=DIRECTION ( 'NONE',  ( -0.5000000000000037748, -0.4999999999999950040, -0.7071067811865484609 ) ) ;
#87979=CARTESIAN_POINT ( 'NONE',  ( -7.500000000000000000, 0.000000000000000000, 0.000000000000000000 ) ) ;
#88143=ORIENTED_EDGE ( 'NONE', *, *, #1107, .T. ) ;
#88176=CARTESIAN_POINT ( 'NONE',  ( 26.99873734152944138, 22.49873734152883387, 1.110912703473986074 ) ) ;
#88236=DIRECTION ( 'NONE',  ( 0.7071067811865512365, 0.7071067811865439090, -0.000000000000000000 ) ) ;
#88322=ORIENTED_EDGE ( 'NONE', *, *, #97283, .T. ) ;
#88384=CARTESIAN_POINT ( 'NONE',  ( 3.424326230466405718, 6.677994727576183287, 1.353258418600855606 ) ) ;
#88433=DIRECTION ( 'NONE',  ( -1.047444401652940164E-14, -1.000000000000000000, -0.000000000000000000 ) ) ;
#88711=EDGE_LOOP ( 'NONE', ( #166525, #80338 ) ) ;
#88744=LINE ( 'NONE', #120074, #183167 ) ;
#88787=CARTESIAN_POINT ( 'NONE',  ( -2.552343178074577779, 7.052343178074668373, 1.110912703473986074 ) ) ;
#88808=VECTOR ( 'NONE', #48939, 1000.000000000000000 ) ;
#88844=EDGE_LOOP ( 'NONE', ( #166757, #170165, #152935, #87570 ) ) ;
#88897=EDGE_CURVE ( 'NONE', #51904, #144525, #74465, .T. ) ;
#89014=DIRECTION ( 'NONE',  ( 0.000000000000000000, 0.8164965809277253683, -0.5773502691896269523 ) ) ;
#89057=VERTEX_POINT ( 'NONE', #189622 ) ;
#89108=DIRECTION ( 'NONE',  ( -0.7071067811865466846, 2.468850131082262977E-15, 0.7071067811865484609 ) ) ;
#89114=ADVANCED_FACE ( 'NONE', ( #173459 ), #175439, .T. ) ;
#89193=VECTOR ( 'NONE', #17635, 1000.000000000000000 ) ;
#89293=EDGE_CURVE ( 'NONE', #9747, #58678, #148648, .T. ) ;
#89538=ORIENTED_EDGE ( 'NONE', *, *, #185853, .T. ) ;
#89590=CARTESIAN_POINT ( 'NONE',  ( -7.052343178074647945, -2.552343178074588437, 1.110912703473986074 ) ) ;
#89603=CARTESIAN_POINT ( 'NONE',  ( -24.99873734152895466, 24.49873734152938454, 4.646446609406721606 ) ) ;
#89709=VERTEX_POINT ( 'NONE', #58091 ) ;
#89912=( NAMED_UNIT ( * ) SI_UNIT ( $, .STERADIAN. ) SOLID_ANGLE_UNIT ( ) );
#90218=EDGE_LOOP ( 'NONE', ( #156982, #20686, #64097, #133304, #4692, #46946 ) ) ;
#90304=CARTESIAN_POINT ( 'NONE',  ( -26.99873734152928506, -22.49873734152901861, 1.110912703473986074 ) ) ;
#90410=CARTESIAN_POINT ( 'NONE',  ( -23.96320343559652599, -18.46320343559629507, 1.818019484660534424 ) ) ;
#90442=VECTOR ( 'NONE', #61151, 1000.000000000000000 ) ;
#90448=( BOUNDED_CURVE ( )  B_SPLINE_CURVE ( 3, ( #53820, #195346, #118501, #180191 ),
 .UNSPECIFIED., .F., .F. ) 
 B_SPLINE_CURVE_WITH_KNOTS ( ( 4, 4 ),
 ( 1.132647296210725241, 2.115944711806983847 ),
 .UNSPECIFIED. ) 
 CURVE ( )  GEOMETRIC_REPRESENTATION_ITEM ( )  RATIONAL_B_SPLINE_CURVE ( ( 1.000000000000000000, 0.9210371567966659789, 0.9210371567966659789, 1.000000000000000000 ) ) 
 REPRESENTATION_ITEM ( '' )  );
#90460=ORIENTED_EDGE ( 'NONE', *, *, #158042, .T. ) ;
#90504=DIRECTION ( 'NONE',  ( 0.000000000000000000, -0.7071067811865483499, 0.7071067811865465735 ) ) ;
#90645=VERTEX_POINT ( 'NONE', #75231 ) ;
#90984=EDGE_CURVE ( 'NONE', #723, #17186, #154058, .T. ) ;
#91072=CARTESIAN_POINT ( 'NONE',  ( 0.000000000000000000, 0.000000000000000000, 0.000000000000000000 ) ) ;
#91221=FACE_OUTER_BOUND ( 'NONE', #127374, .T. ) ;
#91233=CARTESIAN_POINT ( 'NONE',  ( 21.46320343559668231, 20.96320343559617072, 5.353553390593269512 ) ) ;
#91341=DIRECTION ( 'NONE',  ( -0.000000000000000000, -0.000000000000000000, 1.000000000000000000 ) ) ;
#91376=EDGE_CURVE ( 'NONE', #45713, #26126, #192111, .T. ) ;
#91475=FACE_OUTER_BOUND ( 'NONE', #29441, .T. ) ;
#91589=CARTESIAN_POINT ( 'NONE',  ( -20.96320343559653665, -21.46320343559631638, 4.646446609406719830 ) ) ;
#91802=AXIS2_PLACEMENT_3D ( 'NONE', #67115, #37778, #7427 ) ;
#91873=VECTOR ( 'NONE', #10785, 1000.000000000000114 ) ;
#92061=PRODUCT ( 'Impeller Fan Blade Assembly', 'Impeller Fan Blade Assembly', '', ( #82597 ) ) ;
#92199=EDGE_LOOP ( 'NONE', ( #174803, #1902, #157346, #24593 ) ) ;
#92438=ORIENTED_EDGE ( 'NONE', *, *, #193497, .F. ) ;
#92475=DIRECTION ( 'NONE',  ( 0.7071067811865512365, 0.7071067811865439090, -0.000000000000000000 ) ) ;
#92593=DIRECTION ( 'NONE',  ( 0.4999999999999967248, -0.5000000000000019984, -0.7071067811865484609 ) ) ;
#92774=CIRCLE ( 'NONE', #118645, 4.999999999999998224 ) ;
#93013=VERTEX_POINT ( 'NONE', #171733 ) ;
#93254=EDGE_CURVE ( 'NONE', #30636, #75343, #35202, .T. ) ;
#93363=FACE_BOUND ( 'NONE', #13023, .T. ) ;
#93541=FACE_OUTER_BOUND ( 'NONE', #100408, .T. ) ;
#93602=AXIS2_PLACEMENT_3D ( 'NONE', #22862, #38031, #41034 ) ;
#93639=VECTOR ( 'NONE', #60792, 1000.000000000000000 ) ;
#93717=CARTESIAN_POINT ( 'NONE',  ( -7.052343178074620411, 2.552343178074692354, 8.889087296526001936 ) ) ;
#93815=FACE_OUTER_BOUND ( 'NONE', #35739, .T. ) ;
#94075=LINE ( 'NONE', #188103, #159665 ) ;
#94101=EDGE_CURVE ( 'NONE', #17363, #56096, #96914, .T. ) ;
#94276=ORIENTED_EDGE ( 'NONE', *, *, #56725, .T. ) ;
#94427=CARTESIAN_POINT ( 'NONE',  ( 35.00000000000000000, 3.889087296526017479, 8.181980515339454030 ) ) ;
#94539=EDGE_CURVE ( 'NONE', #46039, #138583, #131781, .T. ) ;
#94591=CIRCLE ( 'NONE', #172095, 5.000000000000000888 ) ;
#94749=CARTESIAN_POINT ( 'NONE',  ( -35.00000000000000000, -3.181980515339470905, 8.889087296526001936 ) ) ;
#94772=EDGE_CURVE ( 'NONE', #30159, #141361, #2998, .T. ) ;
#95061=VECTOR ( 'NONE', #21856, 1000.000000000000000 ) ;
#95423=CARTESIAN_POINT ( 'NONE',  ( 30.00000000000000355, -0.3535533905932703447, 5.353553390593268624 ) ) ;
#95459=LINE ( 'NONE', #141958, #72739 ) ;
#95544=CARTESIAN_POINT ( 'NONE',  ( -18.46320343559621691, 23.96320343559658994, 1.818019484660532870 ) ) ;
#95551=DIRECTION ( 'NONE',  ( -0.7071067811865463515, 0.7071067811865487940, -0.000000000000000000 ) ) ;
#95589=DIRECTION ( 'NONE',  ( -0.000000000000000000, 0.7071067811865467956, 0.7071067811865483499 ) ) ;
#95689=DIRECTION ( 'NONE',  ( -0.000000000000000000, -0.7071067811865466846, -0.7071067811865484609 ) ) ;
#95723=ORIENTED_EDGE ( 'NONE', *, *, #117641, .F. ) ;
#95772=VERTEX_POINT ( 'NONE', #87979 ) ;
#95994=DIRECTION ( 'NONE',  ( 0.000000000000000000, 0.7071067811865467956, 0.7071067811865483499 ) ) ;
#96053=CARTESIAN_POINT ( 'NONE',  ( -26.99873734152897242, 22.49873734152939520, 8.889087296526001936 ) ) ;
#96057=CARTESIAN_POINT ( 'NONE',  ( -30.00000000000000355, 0.3535533905932712884, 5.353553390593269512 ) ) ;
#96176=EDGE_CURVE ( 'NONE', #51904, #41517, #137465, .T. ) ;
#96257=VECTOR ( 'NONE', #132784, 1000.000000000000000 ) ;
#96530=PLANE ( 'NONE',  #27082 ) ;
#96548=LINE ( 'NONE', #14009, #101846 ) ;
#96660=EDGE_LOOP ( 'NONE', ( #75898, #146330, #83467, #106435 ) ) ;
#96705=ORIENTED_EDGE ( 'NONE', *, *, #183156, .T. ) ;
#96853=DIRECTION ( 'NONE',  ( -0.7071067811865467956, 2.468850131082262977E-15, 0.7071067811865483499 ) ) ;
#96881=VERTEX_POINT ( 'NONE', #15121 ) ;
#96914=( BOUNDED_CURVE ( )  B_SPLINE_CURVE ( 3, ( #45179, #64316, #139156, #156324 ),
 .UNSPECIFIED., .F., .T. ) 
 B_SPLINE_CURVE_WITH_KNOTS ( ( 4, 4 ),
 ( 5.150538010968861435, 5.257537365396776963 ),
 .UNSPECIFIED. ) 
 CURVE ( )  GEOMETRIC_REPRESENTATION_ITEM ( )  RATIONAL_B_SPLINE_CURVE ( ( 1.000000000000000000, 0.9990461557208837329, 0.9990461557208837329, 1.000000000000000000 ) ) 
 REPRESENTATION_ITEM ( '' )  );
#96937=AXIS2_PLACEMENT_3D ( 'NONE', #112756, #67252, #33943 ) ;
#96947=ADVANCED_FACE ( 'NONE', ( #153625 ), #49436, .T. ) ;
#97163=CYLINDRICAL_SURFACE ( 'NONE', #163138, 4.999999999999999112 ) ;
#97265=ORIENTED_EDGE ( 'NONE', *, *, #134059, .F. ) ;
#97283=EDGE_CURVE ( 'NONE', #171715, #9508, #117612, .T. ) ;
#97390=ORIENTED_EDGE ( 'NONE', *, *, #87134, .T. ) ;
#97638=ORIENTED_EDGE ( 'NONE', *, *, #2501, .T. ) ;
#97685=VERTEX_POINT ( 'NONE', #68569 ) ;
#97757=SHAPE_DEFINITION_REPRESENTATION ( #185759, #8335 ) ;
#97759=EDGE_LOOP ( 'NONE', ( #191905, #172822, #30664, #187232 ) ) ;
#97829=CARTESIAN_POINT ( 'NONE',  ( 18.96320343559671073, 23.46320343559620270, 8.889087296526001936 ) ) ;
#97992=EDGE_LOOP ( 'NONE', ( #6445, #189868, #128321, #34761, #37161 ) ) ;
#98013=DIRECTION ( 'NONE',  ( 0.7071067811865414665, -0.7071067811865536790, -0.000000000000000000 ) ) ;
#98188=CARTESIAN_POINT ( 'NONE',  ( -7.260022482700430047, -2.182060888568185142, 7.889167669754719725 ) ) ;
#98331=AXIS2_PLACEMENT_3D ( 'NONE', #173548, #95689, #83496 ) ;
#98517=CIRCLE ( 'NONE', #37189, 5.000000000000000000 ) ;
#98572=CARTESIAN_POINT ( 'NONE',  ( -21.46320343559653310, -20.96320343559631638, 5.353553390593268624 ) ) ;
#99122=ADVANCED_FACE ( 'NONE', ( #167007, #74983, #44650, #77946 ), #28509, .T. ) ;
#99162=ORIENTED_EDGE ( 'NONE', *, *, #171952, .T. ) ;
#99165=ORIENTED_EDGE ( 'NONE', *, *, #196211, .T. ) ;
#99220=EDGE_LOOP ( 'NONE', ( #198408, #179113, #47714, #9721 ) ) ;
#99242=DIRECTION ( 'NONE',  ( 0.000000000000000000, 0.000000000000000000, 1.000000000000000000 ) ) ;
#99287=VECTOR ( 'NONE', #104443, 1000.000000000000000 ) ;
#99437=EDGE_CURVE ( 'NONE', #191847, #89709, #182172, .T. ) ;
#99441=CARTESIAN_POINT ( 'NONE',  ( 24.99873734152946270, 24.49873734152885874, 5.353553390593270400 ) ) ;
#99442=CARTESIAN_POINT ( 'NONE',  ( 6.791538853603062975, 3.181980515339470905, 8.889087296526001936 ) ) ;
#99526=LINE ( 'NONE', #95544, #37792 ) ;
#99558=CARTESIAN_POINT ( 'NONE',  ( 35.00000000000000000, -3.181980515339468241, 1.110912703473986074 ) ) ;
#99814=CIRCLE ( 'NONE', #60988, 7.500000000000000000 ) ;
#99972=CARTESIAN_POINT ( 'NONE',  ( -3.181980515339156934, 30.00000000000003553, 8.889087296526001936 ) ) ;
#100001=DIRECTION ( 'NONE',  ( -0.4999999999999933387, 0.5000000000000055511, -0.7071067811865484609 ) ) ;
#100113=( BOUNDED_CURVE ( )  B_SPLINE_CURVE ( 3, ( #23387, #115395, #98188, #177083 ),
 .UNSPECIFIED., .F., .T. ) 
 B_SPLINE_CURVE_WITH_KNOTS ( ( 4, 4 ),
 ( 1.570796326794896558, 2.008945357379067431 ),
 .UNSPECIFIED. ) 
 CURVE ( )  GEOMETRIC_REPRESENTATION_ITEM ( )  RATIONAL_B_SPLINE_CURVE ( ( 1.000000000000000000, 0.9840659996946589105, 0.9840659996946589105, 1.000000000000000000 ) ) 
 REPRESENTATION_ITEM ( '' )  );
#100191=ORIENTED_EDGE ( 'NONE', *, *, #15456, .F. ) ;
#100211=DIRECTION ( 'NONE',  ( -0.4999999999999933387, 0.5000000000000055511, -0.7071067811865484609 ) ) ;
#100247=( NAMED_UNIT ( * ) SI_UNIT ( $, .STERADIAN. ) SOLID_ANGLE_UNIT ( ) );
#100408=EDGE_LOOP ( 'NONE', ( #36491, #166352, #140992, #169808 ) ) ;
#100813=EDGE_CURVE ( 'NONE', #97685, #60651, #83920, .T. ) ;
#100957=ORIENTED_EDGE ( 'NONE', *, *, #17615, .F. ) ;
#101164=CARTESIAN_POINT ( 'NONE',  ( 4.962140900324421011, -6.180203150055868733, 3.431593142121016626 ) ) ;
#101197=ADVANCED_FACE ( 'NONE', ( #122365 ), #185043, .T. ) ;
#101215=ORIENTED_EDGE ( 'NONE', *, *, #152294, .T. ) ;
#101267=PLANE ( 'NONE',  #75717 ) ;
#101271=ORIENTED_EDGE ( 'NONE', *, *, #122650, .T. ) ;
#101294=( BOUNDED_CURVE ( )  B_SPLINE_CURVE ( 3, ( #55065, #88384, #23740, #12569 ),
 .UNSPECIFIED., .F., .T. ) 
 B_SPLINE_CURVE_WITH_KNOTS ( ( 4, 4 ),
 ( 2.008945357379066987, 2.115944711806982070 ),
 .UNSPECIFIED. ) 
 CURVE ( )  GEOMETRIC_REPRESENTATION_ITEM ( )  RATIONAL_B_SPLINE_CURVE ( ( 1.000000000000000000, 0.9990461557208837329, 0.9990461557208837329, 1.000000000000000000 ) ) 
 REPRESENTATION_ITEM ( '' )  );
#101353=CARTESIAN_POINT ( 'NONE',  ( -3.889087296525703508, 30.00000000000004263, 8.181980515339454030 ) ) ;
#101441=FACE_OUTER_BOUND ( 'NONE', #90218, .T. ) ;
#101482=EDGE_LOOP ( 'NONE', ( #109039, #162961, #97390, #145523 ) ) ;
#101514=ORIENTED_EDGE ( 'NONE', *, *, #116186, .T. ) ;
#101846=VECTOR ( 'NONE', #74703, 1000.000000000000114 ) ;
#101975=EDGE_CURVE ( 'NONE', #125536, #110145, #180850, .T. ) ;
#102099=CARTESIAN_POINT ( 'NONE',  ( -22.49873734152892624, 26.99873734152936677, 1.110912703473986074 ) ) ;
#102453=DIRECTION ( 'NONE',  ( -0.000000000000000000, 0.7071067811865466846, -0.7071067811865484609 ) ) ;
#102503=DIRECTION ( 'NONE',  ( 0.4999999999999933942, -0.5000000000000055511, 0.7071067811865484609 ) ) ;
#102571=ADVANCED_FACE ( 'NONE', ( #59466 ), #163678, .T. ) ;
#102691=DIRECTION ( 'NONE',  ( 0.5000000000000004441, 0.4999999999999986122, -0.7071067811865481278 ) ) ;
#103057=CARTESIAN_POINT ( 'NONE',  ( 4.273745901508120504, -6.674792076160531273, 4.009310749147818598 ) ) ;
#103203=EDGE_LOOP ( 'NONE', ( #170048, #171287, #191771, #136982, #63719 ) ) ;
#103262=SURFACE_STYLE_USAGE ( .BOTH. , #13247 ) ;
#103350=CARTESIAN_POINT ( 'NONE',  ( 6.674792076160576570, 4.273745901508052114, 4.009310749147818598 ) ) ;
#103367=CARTESIAN_POINT ( 'NONE',  ( 21.99873734152911453, -27.49873734152921045, 1.818019484660534424 ) ) ;
#103419=VERTEX_POINT ( 'NONE', #103962 ) ;
#103503=ORIENTED_EDGE ( 'NONE', *, *, #67374, .F. ) ;
#103622=CARTESIAN_POINT ( 'NONE',  ( 4.273745901508211986, 6.674792076160473542, 5.990689250852167191 ) ) ;
#103704=LINE ( 'NONE', #26877, #90442 ) ;
#103962=CARTESIAN_POINT ( 'NONE',  ( -1.784589286804201480, 7.284589286804282970, 1.818019484660534424 ) ) ;
#104022=ORIENTED_EDGE ( 'NONE', *, *, #154133, .F. ) ;
#104174=ORIENTED_EDGE ( 'NONE', *, *, #171952, .F. ) ;
#104208=CARTESIAN_POINT ( 'NONE',  ( 23.96320343559665389, 18.46320343559613164, 1.818019484660534424 ) ) ;
#104443=DIRECTION ( 'NONE',  ( -0.7071067811865467956, 2.468850131082262977E-15, 0.7071067811865483499 ) ) ;
#104477=DIRECTION ( 'NONE',  ( 0.000000000000000000, -0.7071067811865467956, -0.7071067811865483499 ) ) ;
#104500=FACE_OUTER_BOUND ( 'NONE', #170135, .T. ) ;
#104650=ADVANCED_FACE ( 'NONE', ( #3534 ), #190558, .T. ) ;
#104659=ADVANCED_FACE ( 'NONE', ( #52031 ), #96530, .T. ) ;
#104686=CARTESIAN_POINT ( 'NONE',  ( 23.96320343559640165, -18.46320343559646560, 8.181980515339454030 ) ) ;
#104903=AXIS2_PLACEMENT_3D ( 'NONE', #199552, #91341, #138858 ) ;
#105049=CIRCLE ( 'NONE', #17870, 5.000000000000000000 ) ;
#105202=EDGE_CURVE ( 'NONE', #23611, #26894, #192235, .T. ) ;
#105337=CARTESIAN_POINT ( 'NONE',  ( -6.674792076160553478, -4.273745901508095635, 4.009310749147813269 ) ) ;
#105463=DIRECTION ( 'NONE',  ( -0.5000000000000004441, -0.4999999999999987232, 0.7071067811865482389 ) ) ;
#105481=ORIENTED_EDGE ( 'NONE', *, *, #105202, .T. ) ;
#105651=EDGE_CURVE ( 'NONE', #4246, #9508, #125291, .T. ) ;
#105672=CARTESIAN_POINT ( 'NONE',  ( 3.889087296525994830, -6.412877669190346630, 8.181980515339454030 ) ) ;
#105765=CARTESIAN_POINT ( 'NONE',  ( 18.46320343559638388, -23.96320343559646915, 1.818019484660536200 ) ) ;
#105823=ORIENTED_EDGE ( 'NONE', *, *, #150034, .F. ) ;
#105983=ADVANCED_FACE ( 'NONE', ( #139113 ), #108776, .T. ) ;
#106007=ORIENTED_EDGE ( 'NONE', *, *, #125179, .T. ) ;
#106099=ORIENTED_EDGE ( 'NONE', *, *, #118820, .T. ) ;
#106339=VECTOR ( 'NONE', #10163, 1000.000000000000000 ) ;
#106435=ORIENTED_EDGE ( 'NONE', *, *, #94772, .F. ) ;
#106557=CARTESIAN_POINT ( 'NONE',  ( 0.000000000000000000, 0.000000000000000000, 10.00000000000000000 ) ) ;
#107019=CYLINDRICAL_SURFACE ( 'NONE', #195071, 5.000000000000000888 ) ;
#107366=ORIENTED_EDGE ( 'NONE', *, *, #196169, .T. ) ;
#107392=DIRECTION ( 'NONE',  ( 0.8164965809277261455, 0.000000000000000000, 0.5773502691896257311 ) ) ;
#107411=CARTESIAN_POINT ( 'NONE',  ( 30.00000000000000355, -3.181980515339468241, 1.110912703473986074 ) ) ;
#107422=ORIENTED_EDGE ( 'NONE', *, *, #155322, .F. ) ;
#107511=DIRECTION ( 'NONE',  ( 0.7071067811865466846, -7.406550393246786959E-15, 0.7071067811865484609 ) ) ;
#107520=CARTESIAN_POINT ( 'NONE',  ( 0.000000000000000000, 0.000000000000000000, -20.00000000000000000 ) ) ;
#107532=( BOUNDED_CURVE ( )  B_SPLINE_CURVE ( 3, ( #689, #19850, #2692, #34033 ),
 .UNSPECIFIED., .F., .F. ) 
 B_SPLINE_CURVE_WITH_KNOTS ( ( 4, 4 ),
 ( 5.150538010968860547, 5.257537365396775186 ),
 .UNSPECIFIED. ) 
 CURVE ( )  GEOMETRIC_REPRESENTATION_ITEM ( )  RATIONAL_B_SPLINE_CURVE ( ( 1.000000000000000000, 0.9990461557208837329, 0.9990461557208837329, 1.000000000000000000 ) ) 
 REPRESENTATION_ITEM ( '' )  );
#107792=( BOUNDED_CURVE ( )  B_SPLINE_CURVE ( 3, ( #159891, #55714, #67879, #146714 ),
 .UNSPECIFIED., .F., .T. ) 
 B_SPLINE_CURVE_WITH_KNOTS ( ( 4, 4 ),
 ( 1.025647941782810824, 1.570796326794896780 ),
 .UNSPECIFIED. ) 
 CURVE ( )  GEOMETRIC_REPRESENTATION_ITEM ( )  RATIONAL_B_SPLINE_CURVE ( ( 1.000000000000000000, 0.9753873905749756990, 0.9753873905749756990, 1.000000000000000000 ) ) 
 REPRESENTATION_ITEM ( '' )  );
#107910=VECTOR ( 'NONE', #10463, 1000.000000000000000 ) ;
#107983=EDGE_LOOP ( 'NONE', ( #94276, #106099, #99165, #154359 ) ) ;
#108000=ADVANCED_FACE ( 'NONE', ( #43377 ), #107019, .T. ) ;
#108041=AXIS2_PLACEMENT_3D ( 'NONE', #36597, #131620, #68944 ) ;
#108108=DIRECTION ( 'NONE',  ( 0.4999999999999932276, -0.5000000000000055511, 0.7071067811865484609 ) ) ;
#108190=CARTESIAN_POINT ( 'NONE',  ( -3.181980515339590365, -34.99999999999999289, 1.110912703473986074 ) ) ;
#108206=AXIS2_PLACEMENT_3D ( 'NONE', #47748, #80057, #185258 ) ;
#108246=DIRECTION ( 'NONE',  ( 0.000000000000000000, 0.000000000000000000, 1.000000000000000000 ) ) ;
#108290=CARTESIAN_POINT ( 'NONE',  ( 0.000000000000000000, 0.000000000000000000, 10.00000000000000000 ) ) ;
#108458=ORIENTED_EDGE ( 'NONE', *, *, #184866, .T. ) ;
#108543=FACE_BOUND ( 'NONE', #194261, .T. ) ;
#108719=CYLINDRICAL_SURFACE ( 'NONE', #147557, 5.000000000000000888 ) ;
#108765=PLANE ( 'NONE',  #192481 ) ;
#108776=CYLINDRICAL_SURFACE ( 'NONE', #1198, 5.000000000000000888 ) ;
#109039=ORIENTED_EDGE ( 'NONE', *, *, #132232, .F. ) ;
#109377=ADVANCED_FACE ( 'NONE', ( #1322 ), #47855, .T. ) ;
#109494=EDGE_CURVE ( 'NONE', #175496, #27947, #94591, .T. ) ;
#109514=FACE_OUTER_BOUND ( 'NONE', #68066, .T. ) ;
#109923=( BOUNDED_CURVE ( )  B_SPLINE_CURVE ( 3, ( #46389, #144355, #159519, #35198 ),
 .UNSPECIFIED., .F., .T. ) 
 B_SPLINE_CURVE_WITH_KNOTS ( ( 4, 4 ),
 ( 1.132647296210726351, 1.570796326794896780 ),
 .UNSPECIFIED. ) 
 CURVE ( )  GEOMETRIC_REPRESENTATION_ITEM ( )  RATIONAL_B_SPLINE_CURVE ( ( 1.000000000000000000, 0.9840659996946589105, 0.9840659996946589105, 1.000000000000000000 ) ) 
 REPRESENTATION_ITEM ( '' )  );
#110020=EDGE_CURVE ( 'NONE', #85800, #56096, #90448, .T. ) ;
#110031=ORIENTED_EDGE ( 'NONE', *, *, #109494, .T. ) ;
#110145=VERTEX_POINT ( 'NONE', #73001 ) ;
#110214=ORIENTED_EDGE ( 'NONE', *, *, #150915, .F. ) ;
#110309=CARTESIAN_POINT ( 'NONE',  ( -3.181980515339590365, -34.99999999999999289, 1.110912703473986074 ) ) ;
#110355=ORIENTED_EDGE ( 'NONE', *, *, #184866, .F. ) ;
#110701=CARTESIAN_POINT ( 'NONE',  ( -0.3535533905933752052, -30.00000000000000355, 5.353553390593268624 ) ) ;
#110773=CARTESIAN_POINT ( 'NONE',  ( -22.49873734152892624, 26.99873734152936677, 1.110912703473986074 ) ) ;
#110881=FACE_OUTER_BOUND ( 'NONE', #12531, .T. ) ;
#111104=DIRECTION ( 'NONE',  ( 0.7071067811865467956, 0.000000000000000000, -0.7071067811865483499 ) ) ;
#111346=AXIS2_PLACEMENT_3D ( 'NONE', #106557, #154057, #168234 ) ;
#111358=CARTESIAN_POINT ( 'NONE',  ( -20.96320343559624177, 21.46320343559661126, 5.353553390593268624 ) ) ;
#111514=VECTOR ( 'NONE', #192994, 1000.000000000000000 ) ;
#111587=ORIENTED_EDGE ( 'NONE', *, *, #10842, .F. ) ;
#111592=LINE ( 'NONE', #94427, #88808 ) ;
#111716=DIRECTION ( 'NONE',  ( -0.4999999999999966693, 0.5000000000000019984, 0.7071067811865484609 ) ) ;
#111748=CARTESIAN_POINT ( 'NONE',  ( 0.000000000000000000, 0.000000000000000000, -20.00000000000000000 ) ) ;
#111922=( BOUNDED_CURVE ( )  B_SPLINE_CURVE ( 3, ( #5918, #35273, #50457, #21095 ),
 .UNSPECIFIED., .F., .F. ) 
 B_SPLINE_CURVE_WITH_KNOTS ( ( 4, 4 ),
 ( 1.132647296210726129, 1.570796326794896558 ),
 .UNSPECIFIED. ) 
 CURVE ( )  GEOMETRIC_REPRESENTATION_ITEM ( )  RATIONAL_B_SPLINE_CURVE ( ( 1.000000000000000000, 0.9840659996946589105, 0.9840659996946589105, 1.000000000000000000 ) ) 
 REPRESENTATION_ITEM ( '' )  );
#111946=CARTESIAN_POINT ( 'NONE',  ( 6.791538853603070081, -3.181980515339468241, 1.110912703473986074 ) ) ;
#111963=ORIENTED_EDGE ( 'NONE', *, *, #114488, .F. ) ;
#112026=ORIENTED_EDGE ( 'NONE', *, *, #28043, .F. ) ;
#112103=DIRECTION ( 'NONE',  ( -0.5000000000000004441, -0.4999999999999987232, 0.7071067811865481278 ) ) ;
#112155=EDGE_CURVE ( 'NONE', #33153, #28306, #71744, .T. ) ;
#112174=ORIENTED_EDGE ( 'NONE', *, *, #25449, .F. ) ;
#112223=CARTESIAN_POINT ( 'NONE',  ( -0.3535533905929594267, 30.00000000000000711, 4.646446609406718942 ) ) ;
#112355=FACE_OUTER_BOUND ( 'NONE', #128122, .T. ) ;
#112577=ORIENTED_EDGE ( 'NONE', *, *, #189500, .T. ) ;
#112669=ORIENTED_EDGE ( 'NONE', *, *, #94539, .F. ) ;
#112694=EDGE_CURVE ( 'NONE', #115498, #42832, #910, .T. ) ;
#112733=DIRECTION ( 'NONE',  ( -1.000000000000000000, 0.000000000000000000, -0.000000000000000000 ) ) ;
#112756=CARTESIAN_POINT ( 'NONE',  ( 0.3535533905931707022, -30.00000000000000711, 4.646446609406720718 ) ) ;
#113118=ADVANCED_FACE ( 'NONE', ( #66237 ), #128887, .T. ) ;
#113133=ADVANCED_FACE ( 'NONE', ( #21733 ), #51072, .T. ) ;
#113334=ORIENTED_EDGE ( 'NONE', *, *, #161468, .T. ) ;
#113357=ORIENTED_EDGE ( 'NONE', *, *, #20248, .T. ) ;
#113417=ORIENTED_EDGE ( 'NONE', *, *, #13111, .F. ) ;
#113440=DIRECTION ( 'NONE',  ( 0.7071067811865485719, 0.000000000000000000, 0.7071067811865465735 ) ) ;
#113490=CARTESIAN_POINT ( 'NONE',  ( 2.300691058039425752, -7.143419655154876757, 1.353258418600857382 ) ) ;
#113655=ORIENTED_EDGE ( 'NONE', *, *, #185853, .F. ) ;
#113841=CARTESIAN_POINT ( 'NONE',  ( -35.00000000000000000, -3.889087296526017479, 8.181980515339454030 ) ) ;
#113927=LINE ( 'NONE', #143273, #196167 ) ;
#114053=ADVANCED_FACE ( 'NONE', ( #87398 ), #178424, .T. ) ;
#114277=( BOUNDED_CURVE ( )  B_SPLINE_CURVE ( 3, ( #9574, #181421, #25754, #73250 ),
 .UNSPECIFIED., .F., .T. ) 
 B_SPLINE_CURVE_WITH_KNOTS ( ( 4, 4 ),
 ( 2.008945357379066987, 2.115944711806982070 ),
 .UNSPECIFIED. ) 
 CURVE ( )  GEOMETRIC_REPRESENTATION_ITEM ( )  RATIONAL_B_SPLINE_CURVE ( ( 1.000000000000000000, 0.9990461557208837329, 0.9990461557208837329, 1.000000000000000000 ) ) 
 REPRESENTATION_ITEM ( '' )  );
#114292=ORIENTED_EDGE ( 'NONE', *, *, #168721, .T. ) ;
#114408=CARTESIAN_POINT ( 'NONE',  ( -7.284589286804265207, -1.784589286804211916, 1.818019484660534424 ) ) ;
#114428=AXIS2_PLACEMENT_3D ( 'NONE', #178912, #117218, #161725 ) ;
#114488=EDGE_CURVE ( 'NONE', #19226, #166399, #78169, .T. ) ;
#114653=AXIS2_PLACEMENT_3D ( 'NONE', #110773, #124957, #184645 ) ;
#114656=VERTEX_POINT ( 'NONE', #31691 ) ;
#114876=EDGE_CURVE ( 'NONE', #29557, #81477, #4363, .T. ) ;
#115018=AXIS2_PLACEMENT_3D ( 'NONE', #88176, #54851, #87189 ) ;
#115087=FACE_OUTER_BOUND ( 'NONE', #181269, .T. ) ;
#115338=PRODUCT_DEFINITION ( 'UNKNOWN', '', #188910, #127232 ) ;
#115395=CARTESIAN_POINT ( 'NONE',  ( -7.500000000000001776, -1.104226503365435486, 6.811333284551973399 ) ) ;
#115462=ORIENTED_EDGE ( 'NONE', *, *, #97283, .F. ) ;
#115498=VERTEX_POINT ( 'NONE', #188357 ) ;
#115632=DIRECTION ( 'NONE',  ( 0.000000000000000000, -0.7071067811865483499, 0.7071067811865465735 ) ) ;
#115639=CARTESIAN_POINT ( 'NONE',  ( -7.284589286804255437, 1.784589286804319386, 8.181980515339454030 ) ) ;
#115775=ORIENTED_EDGE ( 'NONE', *, *, #105651, .F. ) ;
#115887=EDGE_LOOP ( 'NONE', ( #41995, #194728, #145934, #180658 ) ) ;
#116131=AXIS2_PLACEMENT_3D ( 'NONE', #83148, #39652, #191334 ) ;
#116186=EDGE_CURVE ( 'NONE', #191800, #81477, #133660, .T. ) ;
#116391=CARTESIAN_POINT ( 'NONE',  ( 1.697796032038702219, -7.741785448087965094, 5.990689250852171632 ) ) ;
#116539=CARTESIAN_POINT ( 'NONE',  ( 4.500000000000000000, 0.000000000000000000, -20.00000000000000000 ) ) ;
#116669=ORIENTED_EDGE ( 'NONE', *, *, #165696, .F. ) ;
#116778=CARTESIAN_POINT ( 'NONE',  ( 7.052343178074679031, 2.552343178074557350, 1.110912703473986074 ) ) ;
#116832=VERTEX_POINT ( 'NONE', #63777 ) ;
#116846=CARTESIAN_POINT ( 'NONE',  ( 30.00000000000000355, 0.3535533905932735643, 4.646446609406718942 ) ) ;
#116929=FACE_OUTER_BOUND ( 'NONE', #169156, .T. ) ;
#117169=ADVANCED_BREP_SHAPE_REPRESENTATION ( '', ( #79223, #82054 ), #65912 ) ;
#117218=DIRECTION ( 'NONE',  ( 0.5000000000000002220, 0.4999999999999985012, -0.7071067811865483499 ) ) ;
#117243=( BOUNDED_CURVE ( )  B_SPLINE_CURVE ( 3, ( #54842, #103350, #165029, #25535 ),
 .UNSPECIFIED., .F., .F. ) 
 B_SPLINE_CURVE_WITH_KNOTS ( ( 4, 4 ),
 ( 1.025647941782811046, 2.008945357379067431 ),
 .UNSPECIFIED. ) 
 CURVE ( )  GEOMETRIC_REPRESENTATION_ITEM ( )  RATIONAL_B_SPLINE_CURVE ( ( 1.000000000000000000, 0.9210371567966664230, 0.9210371567966664230, 1.000000000000000000 ) ) 
 REPRESENTATION_ITEM ( '' )  );
#117523=CARTESIAN_POINT ( 'NONE',  ( -21.46320343559653665, -25.04568634023494056, 8.240304736541402164 ) ) ;
#117612=( BOUNDED_CURVE ( )  B_SPLINE_CURVE ( 3, ( #184964, #142430, #155617, #172787 ),
 .UNSPECIFIED., .F., .F. ) 
 B_SPLINE_CURVE_WITH_KNOTS ( ( 4, 4 ),
 ( 5.150538010968860547, 5.257537365396776075 ),
 .UNSPECIFIED. ) 
 CURVE ( )  GEOMETRIC_REPRESENTATION_ITEM ( )  RATIONAL_B_SPLINE_CURVE ( ( 1.000000000000000000, 0.9990461557208837329, 0.9990461557208837329, 1.000000000000000000 ) ) 
 REPRESENTATION_ITEM ( '' )  );
#117622=CARTESIAN_POINT ( 'NONE',  ( 30.00000000000000355, 0.3535533905932755627, 4.646446609406720718 ) ) ;
#117641=EDGE_CURVE ( 'NONE', #159190, #103419, #124445, .T. ) ;
#117681=DIRECTION ( 'NONE',  ( -0.7071067811865463515, 0.7071067811865487940, -0.000000000000000000 ) ) ;
#117744=CIRCLE ( 'NONE', #72574, 5.000000000000000888 ) ;
#118141=CARTESIAN_POINT ( 'NONE',  ( -2.300691058039380454, 7.143419655154890968, 1.353258418600854274 ) ) ;
#118234=CARTESIAN_POINT ( 'NONE',  ( 22.49873734152911453, -26.99873734152921045, 1.110912703473986074 ) ) ;
#118501=CARTESIAN_POINT ( 'NONE',  ( -4.273745901508164025, -6.674792076160507293, 5.990689250852175185 ) ) ;
#118504=ORIENTED_EDGE ( 'NONE', *, *, #37374, .T. ) ;
#118596=ORIENTED_EDGE ( 'NONE', *, *, #37272, .T. ) ;
#118645=AXIS2_PLACEMENT_3D ( 'NONE', #151929, #45740, #107392 ) ;
#118662=DIRECTION ( 'NONE',  ( 0.7071067811865467956, 0.000000000000000000, 0.7071067811865483499 ) ) ;
#118820=EDGE_CURVE ( 'NONE', #103419, #18224, #160115, .T. ) ;
#118873=LINE ( 'NONE', #180557, #87361 ) ;
#119121=CARTESIAN_POINT ( 'NONE',  ( 22.49873734152949112, 26.99873734152889782, 8.889087296526001936 ) ) ;
#119184=DIRECTION ( 'NONE',  ( 0.8164965809277249242, 0.000000000000000000, -0.5773502691896271743 ) ) ;
#119376=ORIENTED_EDGE ( 'NONE', *, *, #3003, .T. ) ;
#119460=CARTESIAN_POINT ( 'NONE',  ( -23.96320343559627375, 18.46320343559663257, 8.181980515339454030 ) ) ;
#119620=DIRECTION ( 'NONE',  ( 0.000000000000000000, 0.7071067811865483499, 0.7071067811865465735 ) ) ;
#119864=CARTESIAN_POINT ( 'NONE',  ( -35.00000000000000000, 3.181980515339468241, 1.110912703473986074 ) ) ;
#119923=ADVANCED_FACE ( 'NONE', ( #133031 ), #7672, .F. ) ;
#120074=CARTESIAN_POINT ( 'NONE',  ( -26.99873734152928506, -22.49873734152901861, 1.110912703473986074 ) ) ;
#120197=DIRECTION ( 'NONE',  ( 0.5000000000000002220, 0.4999999999999985012, -0.7071067811865483499 ) ) ;
#120314=CARTESIAN_POINT ( 'NONE',  ( -21.46320343559653665, -20.96320343559631638, 5.353553390593268624 ) ) ;
#120508=CARTESIAN_POINT ( 'NONE',  ( 3.889087296526381632, 34.99999999999996447, 1.818019484660534424 ) ) ;
#120577=AXIS2_PLACEMENT_3D ( 'NONE', #174183, #189355, #64996 ) ;
#120611=CARTESIAN_POINT ( 'NONE',  ( 3.181980515339446924, -6.791538853603077186, 8.889087296526001936 ) ) ;
#120670=VERTEX_POINT ( 'NONE', #134041 ) ;
#120749=DIRECTION ( 'NONE',  ( 1.000000000000000000, 0.000000000000000000, 0.000000000000000000 ) ) ;
#120835=EDGE_CURVE ( 'NONE', #198713, #29557, #103704, .T. ) ;
#121146=AXIS2_PLACEMENT_3D ( 'NONE', #118234, #70728, #149561 ) ;
#121162=ADVANCED_FACE ( 'NONE', ( #91475 ), #58196, .F. ) ;
#121184=CIRCLE ( 'NONE', #147028, 4.999999999999998224 ) ;
#121428=ORIENTED_EDGE ( 'NONE', *, *, #6906, .T. ) ;
#121461=EDGE_LOOP ( 'NONE', ( #51781, #32252, #18660, #62966 ) ) ;
#121593=DIRECTION ( 'NONE',  ( -1.000000000000000000, -0.000000000000000000, -0.000000000000000000 ) ) ;
#121823=ADVANCED_FACE ( 'NONE', ( #101441 ), #193476, .T. ) ;
#121903=ORIENTED_EDGE ( 'NONE', *, *, #139056, .T. ) ;
#121905=CARTESIAN_POINT ( 'NONE',  ( 30.00000000000000355, -0.3535533905932729537, 5.353553390593267736 ) ) ;
#121967=STYLED_ITEM ( 'NONE', ( #75724 ), #79223 ) ;
#122157=VERTEX_POINT ( 'NONE', #130782 ) ;
#122164=ORIENTED_EDGE ( 'NONE', *, *, #16838, .T. ) ;
#122363=ORIENTED_EDGE ( 'NONE', *, *, #154133, .T. ) ;
#122365=FACE_OUTER_BOUND ( 'NONE', #121461, .T. ) ;
#122452=CARTESIAN_POINT ( 'NONE',  ( -21.99873734152892268, 27.49873734152935967, 1.818019484660534424 ) ) ;
#122466=VECTOR ( 'NONE', #146595, 1000.000000000000000 ) ;
#122650=EDGE_CURVE ( 'NONE', #30636, #120670, #177959, .T. ) ;
#122870=ORIENTED_EDGE ( 'NONE', *, *, #156994, .T. ) ;
#123068=CARTESIAN_POINT ( 'NONE',  ( 0.3535533905931536602, -35.00000000000000000, 4.646446609406721606 ) ) ;
#123075=VERTEX_POINT ( 'NONE', #84916 ) ;
#123454=EDGE_CURVE ( 'NONE', #28306, #50238, #1251, .T. ) ;
#123466=DIRECTION ( 'NONE',  ( -0.5000000000000014433, -0.4999999999999996114, -0.7071067811865467956 ) ) ;
#123563=CARTESIAN_POINT ( 'NONE',  ( 21.99873734152911453, -27.49873734152921045, 1.818019484660534424 ) ) ;
#123694=FACE_OUTER_BOUND ( 'NONE', #52893, .T. ) ;
#123695=DIRECTION ( 'NONE',  ( 0.000000000000000000, -0.7071067811865467956, 0.7071067811865483499 ) ) ;
#124212=SURFACE_STYLE_USAGE ( .BOTH. , #77715 ) ;
#124445=LINE ( 'NONE', #122452, #171113 ) ;
#124573=CARTESIAN_POINT ( 'NONE',  ( 30.00000000000000355, -3.889087296526014814, 1.818019484660534424 ) ) ;
#124584=VECTOR ( 'NONE', #56871, 1000.000000000000000 ) ;
#124777=ORIENTED_EDGE ( 'NONE', *, *, #184979, .F. ) ;
#124957=DIRECTION ( 'NONE',  ( 0.5000000000000049960, 0.4999999999999962252, -0.7071067811865466846 ) ) ;
#125061=CARTESIAN_POINT ( 'NONE',  ( -4.273745901508076983, 6.674792076160563248, 4.009310749147818598 ) ) ;
#125179=EDGE_CURVE ( 'NONE', #180340, #185456, #99814, .T. ) ;
#125266=CARTESIAN_POINT ( 'NONE',  ( 20.96320343559639454, -21.46320343559646560, 5.353553390593270400 ) ) ;
#125291=( BOUNDED_CURVE ( )  B_SPLINE_CURVE ( 3, ( #177402, #148051, #162209, #74204 ),
 .UNSPECIFIED., .F., .F. ) 
 B_SPLINE_CURVE_WITH_KNOTS ( ( 4, 4 ),
 ( 1.570796326794896558, 2.115944711806982959 ),
 .UNSPECIFIED. ) 
 CURVE ( )  GEOMETRIC_REPRESENTATION_ITEM ( )  RATIONAL_B_SPLINE_CURVE ( ( 1.000000000000000000, 0.9753873905749756990, 0.9753873905749756990, 1.000000000000000000 ) ) 
 REPRESENTATION_ITEM ( '' )  );
#125481=DIRECTION ( 'NONE',  ( 0.8164965809277261455, -6.938893903907231336E-16, 0.5773502691896253980 ) ) ;
#125489=CARTESIAN_POINT ( 'NONE',  ( 3.889087296526082316, 6.412877669190294228, 1.818019484660534424 ) ) ;
#125536=VERTEX_POINT ( 'NONE', #161882 ) ;
#125567=CARTESIAN_POINT ( 'NONE',  ( -3.181980515339492221, -6.791538853603052317, 1.110912703473986074 ) ) ;
#125644=ORIENTED_EDGE ( 'NONE', *, *, #35339, .T. ) ;
#126396=EDGE_CURVE ( 'NONE', #95772, #90645, #154672, .T. ) ;
#126704=CARTESIAN_POINT ( 'NONE',  ( 0.000000000000000000, 0.000000000000000000, -20.00000000000000000 ) ) ;
#126710=EDGE_CURVE ( 'NONE', #128792, #15917, #38296, .T. ) ;
#126870=DIRECTION ( 'NONE',  ( -0.4999999999999967248, 0.5000000000000019984, 0.7071067811865485719 ) ) ;
#127061=DIRECTION ( 'NONE',  ( -0.7071067811865467956, 7.406550393246786959E-15, -0.7071067811865483499 ) ) ;
#127109=CARTESIAN_POINT ( 'NONE',  ( -3.889087296526037463, -6.412877669190318208, 1.818019484660534424 ) ) ;
#127189=CARTESIAN_POINT ( 'NONE',  ( 3.181980515339365656, -30.00000000000001776, 8.889087296526001936 ) ) ;
#127232=PRODUCT_DEFINITION_CONTEXT ( 'detailed design', #50677, 'design' ) ;
#127374=EDGE_LOOP ( 'NONE', ( #110355, #184417, #138527, #84701 ) ) ;
#127599=ORIENTED_EDGE ( 'NONE', *, *, #86511, .T. ) ;
#127650=AXIS2_PLACEMENT_3D ( 'NONE', #29203, #76674, #137354 ) ;
#127807=CARTESIAN_POINT ( 'NONE',  ( 23.46320343559640165, -18.96320343559646204, 8.889087296526001936 ) ) ;
#127830=ORIENTED_EDGE ( 'NONE', *, *, #145930, .F. ) ;
#127846=CIRCLE ( 'NONE', #31031, 4.999999999999999112 ) ;
#127929=EDGE_LOOP ( 'NONE', ( #195441, #167384, #122363, #184811, #188282, #89538, #170664, #136840, #196358, #128609, #188832, #71897 ) ) ;
#127996=ORIENTED_EDGE ( 'NONE', *, *, #35339, .F. ) ;
#128122=EDGE_LOOP ( 'NONE', ( #25131, #138470, #104174, #77367 ) ) ;
#128228=LINE ( 'NONE', #83713, #20991 ) ;
#128314=VECTOR ( 'NONE', #60638, 1000.000000000000000 ) ;
#128321=ORIENTED_EDGE ( 'NONE', *, *, #185673, .T. ) ;
#128355=EDGE_CURVE ( 'NONE', #191800, #198713, #199998, .T. ) ;
#128448=CARTESIAN_POINT ( 'NONE',  ( -1.697796032038755287, -7.741785448087954435, 4.009310749147816821 ) ) ;
#128609=ORIENTED_EDGE ( 'NONE', *, *, #94539, .T. ) ;
#128762=ORIENTED_EDGE ( 'NONE', *, *, #174237, .T. ) ;
#128792=VERTEX_POINT ( 'NONE', #30703 ) ;
#128887=CYLINDRICAL_SURFACE ( 'NONE', #181931, 5.000000000000000888 ) ;
#129254=CARTESIAN_POINT ( 'NONE',  ( -26.99873734152897242, 22.49873734152939520, 8.889087296526001936 ) ) ;
#129302=CARTESIAN_POINT ( 'NONE',  ( -35.00000000000000000, 3.181980515339468241, 1.110912703473986074 ) ) ;
#129609=EDGE_CURVE ( 'NONE', #110145, #115498, #15975, .T. ) ;
#129810=VERTEX_POINT ( 'NONE', #66990 ) ;
#129876=CARTESIAN_POINT ( 'NONE',  ( 0.3535533905931680931, -30.00000000000000355, 4.646446609406719830 ) ) ;
#130325=CARTESIAN_POINT ( 'NONE',  ( 18.96320343559638388, -23.46320343559646560, 1.110912703473986074 ) ) ;
#130520=ORIENTED_EDGE ( 'NONE', *, *, #93254, .F. ) ;
#130564=AXIS2_PLACEMENT_3D ( 'NONE', #38554, #100211, #40554 ) ;
#130572=( GEOMETRIC_REPRESENTATION_CONTEXT ( 3 ) GLOBAL_UNCERTAINTY_ASSIGNED_CONTEXT ( ( #161139 ) ) GLOBAL_UNIT_ASSIGNED_CONTEXT ( ( #150771, #134608, #72939 ) ) REPRESENTATION_CONTEXT ( 'NONE', 'WORKASPACE' ) );
#130687=DIRECTION ( 'NONE',  ( 0.000000000000000000, 0.7071067811865466846, 0.7071067811865484609 ) ) ;
#130782=CARTESIAN_POINT ( 'NONE',  ( -0.3535533905929095222, 35.00000000000000000, 4.646446609406721606 ) ) ;
#130824=EDGE_LOOP ( 'NONE', ( #111963, #178898, #57395, #35131 ) ) ;
#130858=AXIS2_PLACEMENT_3D ( 'NONE', #103367, #149866, #150874 ) ;
#130941=AXIS2_PLACEMENT_3D ( 'NONE', #110309, #2136, #80957 ) ;
#131122=EDGE_LOOP ( 'NONE', ( #77575, #145782, #113357, #112669 ) ) ;
#131249=PLANE ( 'NONE',  #153204 ) ;
#131620=DIRECTION ( 'NONE',  ( 0.000000000000000000, -0.7071067811865466846, 0.7071067811865484609 ) ) ;
#131781=( BOUNDED_CURVE ( )  B_SPLINE_CURVE ( 3, ( #80990, #80006, #142665, #4144 ),
 .UNSPECIFIED., .F., .T. ) 
 B_SPLINE_CURVE_WITH_KNOTS ( ( 4, 4 ),
 ( 2.008945357379066987, 2.115944711806982070 ),
 .UNSPECIFIED. ) 
 CURVE ( )  GEOMETRIC_REPRESENTATION_ITEM ( )  RATIONAL_B_SPLINE_CURVE ( ( 1.000000000000000000, 0.9990461557208837329, 0.9990461557208837329, 1.000000000000000000 ) ) 
 REPRESENTATION_ITEM ( '' )  );
#131792=CARTESIAN_POINT ( 'NONE',  ( 6.551653823223136719, 3.660253528765625486, 8.410814283099844246 ) ) ;
#132232=EDGE_CURVE ( 'NONE', #89057, #18224, #38376, .T. ) ;
#132521=CARTESIAN_POINT ( 'NONE',  ( 7.284589286804261654, -1.784589286804270980, 8.181980515339454030 ) ) ;
#132628=VERTEX_POINT ( 'NONE', #83857 ) ;
#132662=EDGE_LOOP ( 'NONE', ( #135631, #187655, #72170, #96705, #178806, #107422 ) ) ;
#132749=ORIENTED_EDGE ( 'NONE', *, *, #196169, .F. ) ;
#132784=DIRECTION ( 'NONE',  ( -0.7071067811865561215, -0.7071067811865389130, -0.000000000000000000 ) ) ;
#132933=EDGE_CURVE ( 'NONE', #122157, #64689, #82470, .T. ) ;
#133031=FACE_OUTER_BOUND ( 'NONE', #198500, .T. ) ;
#133304=ORIENTED_EDGE ( 'NONE', *, *, #31820, .T. ) ;
#133397=CARTESIAN_POINT ( 'NONE',  ( -3.181980515339573046, -29.99999999999998934, 1.110912703473986074 ) ) ;
#133545=EDGE_CURVE ( 'NONE', #153939, #79638, #121184, .T. ) ;
#133660=LINE ( 'NONE', #9330, #143212 ) ;
#133752=VERTEX_POINT ( 'NONE', #168680 ) ;
#134041=CARTESIAN_POINT ( 'NONE',  ( 7.052343178074679031, 2.552343178074557350, 1.110912703473986074 ) ) ;
#134059=EDGE_CURVE ( 'NONE', #152327, #125536, #96548, .T. ) ;
#134066=AXIS2_PLACEMENT_3D ( 'NONE', #44169, #42187, #167515 ) ;
#134165=ADVANCED_FACE ( 'NONE', ( #65227 ), #136367, .F. ) ;
#134289=LINE ( 'NONE', #119121, #4830 ) ;
#134405=CARTESIAN_POINT ( 'NONE',  ( 7.052343178074640839, -2.552343178074650609, 8.889087296526001936 ) ) ;
#134608=( NAMED_UNIT ( * ) PLANE_ANGLE_UNIT ( ) SI_UNIT ( $, .RADIAN. ) );
#134762=EDGE_LOOP ( 'NONE', ( #181848, #13033, #163134, #62098 ) ) ;
#134859=EDGE_LOOP ( 'NONE', ( #103503, #190433, #46709, #70200 ) ) ;
#135311=CARTESIAN_POINT ( 'NONE',  ( -24.49873734152895111, 24.99873734152937743, 5.353553390593268624 ) ) ;
#135350=EDGE_CURVE ( 'NONE', #80087, #165429, #168850, .T. ) ;
#135372=EDGE_LOOP ( 'NONE', ( #184079, #73182 ) ) ;
#135441=FILL_AREA_STYLE ('',( #182929 ) ) ;
#135510=DIRECTION ( 'NONE',  ( 0.5000000000000037748, 0.4999999999999950595, 0.7071067811865484609 ) ) ;
#135631=ORIENTED_EDGE ( 'NONE', *, *, #101975, .T. ) ;
#135840=DIRECTION ( 'NONE',  ( 0.000000000000000000, -0.8164965809277234809, -0.5773502691896292838 ) ) ;
#135922=( BOUNDED_CURVE ( )  B_SPLINE_CURVE ( 3, ( #125489, #142633, #187186, #19309 ),
 .UNSPECIFIED., .F., .F. ) 
 B_SPLINE_CURVE_WITH_KNOTS ( ( 4, 4 ),
 ( 1.025647941782811046, 2.008945357379067431 ),
 .UNSPECIFIED. ) 
 CURVE ( )  GEOMETRIC_REPRESENTATION_ITEM ( )  RATIONAL_B_SPLINE_CURVE ( ( 1.000000000000000000, 0.9210371567966664230, 0.9210371567966664230, 1.000000000000000000 ) ) 
 REPRESENTATION_ITEM ( '' )  );
#135993=DIRECTION ( 'NONE',  ( 0.8164965809277261455, 0.000000000000000000, 0.5773502691896257311 ) ) ;
#136231=EDGE_CURVE ( 'NONE', #37612, #89057, #166092, .T. ) ;
#136367=PLANE ( 'NONE',  #127650 ) ;
#136726=ORIENTED_EDGE ( 'NONE', *, *, #160293, .F. ) ;
#136840=ORIENTED_EDGE ( 'NONE', *, *, #37272, .F. ) ;
#136968=ORIENTED_EDGE ( 'NONE', *, *, #132232, .T. ) ;
#136982=ORIENTED_EDGE ( 'NONE', *, *, #143563, .T. ) ;
#137115=CIRCLE ( 'NONE', #179141, 5.000000000000000000 ) ;
#137261=ORIENTED_EDGE ( 'NONE', *, *, #14195, .T. ) ;
#137354=DIRECTION ( 'NONE',  ( 0.000000000000000000, -0.7071067811865483499, -0.7071067811865465735 ) ) ;
#137445=EDGE_CURVE ( 'NONE', #138583, #196688, #68207, .T. ) ;
#137465=LINE ( 'NONE', #41499, #106339 ) ;
#137564=LINE ( 'NONE', #138553, #167284 ) ;
#137794=ADVANCED_FACE ( 'NONE', ( #115087 ), #131249, .T. ) ;
#137866=DIRECTION ( 'NONE',  ( -0.000000000000000000, 0.7071067811865483499, 0.7071067811865467956 ) ) ;
#137957=ORIENTED_EDGE ( 'NONE', *, *, #118820, .F. ) ;
#138073=ORIENTED_EDGE ( 'NONE', *, *, #145930, .T. ) ;
#138076=DIRECTION ( 'NONE',  ( 0.000000000000000000, -0.7071067811865466846, 0.7071067811865484609 ) ) ;
#138109=AXIS2_PLACEMENT_3D ( 'NONE', #90304, #9504, #150008 ) ;
#138111=FACE_OUTER_BOUND ( 'NONE', #156050, .T. ) ;
#138470=ORIENTED_EDGE ( 'NONE', *, *, #181979, .T. ) ;
#138527=ORIENTED_EDGE ( 'NONE', *, *, #86587, .F. ) ;
#138553=CARTESIAN_POINT ( 'NONE',  ( 22.49873734152911453, -26.99873734152921045, 1.110912703473986074 ) ) ;
#138583=VERTEX_POINT ( 'NONE', #75551 ) ;
#138858=DIRECTION ( 'NONE',  ( 1.000000000000000000, 0.000000000000000000, 0.000000000000000000 ) ) ;
#138898=CARTESIAN_POINT ( 'NONE',  ( 0.3535533905936371069, 34.99999999999999289, 5.353553390593268624 ) ) ;
#139056=EDGE_CURVE ( 'NONE', #27352, #166707, #78871, .T. ) ;
#139060=ORIENTED_EDGE ( 'NONE', *, *, #3105, .T. ) ;
#139113=FACE_OUTER_BOUND ( 'NONE', #134859, .T. ) ;
#139134=ORIENTED_EDGE ( 'NONE', *, *, #189500, .F. ) ;
#139156=CARTESIAN_POINT ( 'NONE',  ( -2.044528755335720316, -7.220908937440006170, 8.410814283099840694 ) ) ;
#139323=PLANE ( 'NONE',  #157313 ) ;
#139430=CIRCLE ( 'NONE', #10292, 7.500000000000000000 ) ;
#139505=CARTESIAN_POINT ( 'NONE',  ( 18.46320343559671429, 23.96320343559620625, 8.181980515339455806 ) ) ;
#139516=ORIENTED_EDGE ( 'NONE', *, *, #10280, .T. ) ;
#139695=CARTESIAN_POINT ( 'NONE',  ( -18.46320343559621691, 23.96320343559658994, 1.818019484660534424 ) ) ;
#139833=DIRECTION ( 'NONE',  ( 0.7071067811865483499, 0.000000000000000000, -0.7071067811865465735 ) ) ;
#139917=EDGE_CURVE ( 'NONE', #141361, #51904, #14059, .T. ) ;
#140039=PLANE ( 'NONE',  #73245 ) ;
#140363=ORIENTED_EDGE ( 'NONE', *, *, #162333, .F. ) ;
#140571=CARTESIAN_POINT ( 'NONE',  ( 3.889087296525912674, -30.00000000000002132, 8.181980515339454030 ) ) ;
#140646=FACE_OUTER_BOUND ( 'NONE', #52207, .T. ) ;
#140698=CYLINDRICAL_SURFACE ( 'NONE', #27493, 5.000000000000000888 ) ;
#140992=ORIENTED_EDGE ( 'NONE', *, *, #36780, .T. ) ;
#141068=EDGE_CURVE ( 'NONE', #84463, #23611, #109923, .T. ) ;
#141249=DIRECTION ( 'NONE',  ( 0.5000000000000036637, 0.4999999999999949485, 0.7071067811865484609 ) ) ;
#141361=VERTEX_POINT ( 'NONE', #127189 ) ;
#141958=CARTESIAN_POINT ( 'NONE',  ( -27.49873734152928151, -21.99873734152901861, 1.818019484660534424 ) ) ;
#142039=CARTESIAN_POINT ( 'NONE',  ( -7.284589286804255437, 1.784589286804319386, 8.181980515339454030 ) ) ;
#142115=CARTESIAN_POINT ( 'NONE',  ( -6.412877669190332419, -3.889087296526017479, 8.181980515339454030 ) ) ;
#142206=CARTESIAN_POINT ( 'NONE',  ( -1.784589286804201480, 7.284589286804282970, 1.818019484660534424 ) ) ;
#142430=CARTESIAN_POINT ( 'NONE',  ( -6.677994727576217926, -3.424326230466338661, 8.646741581399133736 ) ) ;
#142539=ORIENTED_EDGE ( 'NONE', *, *, #6876, .F. ) ;
#142633=CARTESIAN_POINT ( 'NONE',  ( 1.697796032038806358, 7.741785448087941113, 4.009310749147818598 ) ) ;
#142665=CARTESIAN_POINT ( 'NONE',  ( -6.551653823223139383, 3.660253528765621045, 1.589185716900141543 ) ) ;
#142848=DIRECTION ( 'NONE',  ( -1.000000000000000000, -0.000000000000000000, -0.000000000000000000 ) ) ;
#143077=DIRECTION ( 'NONE',  ( 0.000000000000000000, -0.7071067811865483499, 0.7071067811865465735 ) ) ;
#143212=VECTOR ( 'NONE', #149829, 1000.000000000000000 ) ;
#143273=CARTESIAN_POINT ( 'NONE',  ( -24.99873734152929217, -24.49873734152903282, 5.353553390593268624 ) ) ;
#143354=DIRECTION ( 'NONE',  ( 0.4999999999999932832, -0.5000000000000055511, 0.7071067811865483499 ) ) ;
#143389=CARTESIAN_POINT ( 'NONE',  ( -7.500000000000000000, 0.000000000000000000, 10.00000000000000000 ) ) ;
#143465=AXIS2_PLACEMENT_3D ( 'NONE', #162125, #35780, #20607 ) ;
#143466=DIRECTION ( 'NONE',  ( 0.7071067811865467956, -7.406550393246788537E-15, 0.7071067811865483499 ) ) ;
#143521=AXIS2_PLACEMENT_3D ( 'NONE', #162830, #135510, #196199 ) ;
#143563=EDGE_CURVE ( 'NONE', #80087, #52906, #134289, .T. ) ;
#143704=CIRCLE ( 'NONE', #156567, 5.000000000000000888 ) ;
#143908=ORIENTED_EDGE ( 'NONE', *, *, #184085, .T. ) ;
#144030=ORIENTED_EDGE ( 'NONE', *, *, #117641, .T. ) ;
#144035=CARTESIAN_POINT ( 'NONE',  ( 18.46320343559671429, 23.96320343559620625, 8.181980515339454030 ) ) ;
#144038=DIRECTION ( 'NONE',  ( 0.000000000000000000, -0.8164965809277251463, 0.5773502691896268413 ) ) ;
#144315=AXIS2_PLACEMENT_3D ( 'NONE', #189949, #19109, #111104 ) ;
#144353=CARTESIAN_POINT ( 'NONE',  ( 24.99873734152912519, -24.49873734152920690, 4.646446609406722494 ) ) ;
#144355=CARTESIAN_POINT ( 'NONE',  ( 7.260022482700430935, -2.182060888568182033, 2.110832330245268729 ) ) ;
#144525=VERTEX_POINT ( 'NONE', #123068 ) ;
#144552=CARTESIAN_POINT ( 'NONE',  ( 0.3535533905936372179, 34.99999999999999289, 5.353553390593270400 ) ) ;
#144635=VERTEX_POINT ( 'NONE', #16899 ) ;
#144751=( NAMED_UNIT ( * ) PLANE_ANGLE_UNIT ( ) SI_UNIT ( $, .RADIAN. ) );
#144840=LINE ( 'NONE', #6324, #179214 ) ;
#145175=DIRECTION ( 'NONE',  ( -6.938893903907227392E-16, -0.7071067811865483499, -0.7071067811865465735 ) ) ;
#145326=EDGE_CURVE ( 'NONE', #177515, #86241, #3699, .T. ) ;
#145393=ORIENTED_EDGE ( 'NONE', *, *, #175772, .T. ) ;
#145523=ORIENTED_EDGE ( 'NONE', *, *, #196211, .F. ) ;
#145634=ORIENTED_EDGE ( 'NONE', *, *, #187016, .F. ) ;
#145782=ORIENTED_EDGE ( 'NONE', *, *, #167192, .T. ) ;
#145864=FACE_OUTER_BOUND ( 'NONE', #75757, .T. ) ;
#145930=EDGE_CURVE ( 'NONE', #4626, #45713, #14524, .T. ) ;
#145934=ORIENTED_EDGE ( 'NONE', *, *, #99437, .T. ) ;
#146330=ORIENTED_EDGE ( 'NONE', *, *, #88897, .F. ) ;
#146352=CARTESIAN_POINT ( 'NONE',  ( 23.96320343559665389, 18.46320343559613164, 1.818019484660535090 ) ) ;
#146533=DIRECTION ( 'NONE',  ( 0.8164965809277261455, 0.000000000000000000, 0.5773502691896257311 ) ) ;
#146595=DIRECTION ( 'NONE',  ( -0.7071067811865561215, -0.7071067811865389130, -0.000000000000000000 ) ) ;
#146714=CARTESIAN_POINT ( 'NONE',  ( 7.500000000000000000, 9.184850993605147944E-16, 5.707106781186540800 ) ) ;
#146847=CARTESIAN_POINT ( 'NONE',  ( 30.00000000000000355, 3.889087296526017479, 8.181980515339454030 ) ) ;
#146857=FACE_OUTER_BOUND ( 'NONE', #11543, .T. ) ;
#147028=AXIS2_PLACEMENT_3D ( 'NONE', #86872, #120197, #146533 ) ;
#147196=CYLINDRICAL_SURFACE ( 'NONE', #188682, 5.000000000000000888 ) ;
#147431=DIRECTION ( 'NONE',  ( -0.7071067811865466846, 2.468850131082262583E-15, 0.7071067811865484609 ) ) ;
#147508=EDGE_CURVE ( 'NONE', #185456, #180340, #163296, .T. ) ;
#147557=AXIS2_PLACEMENT_3D ( 'NONE', #110701, #2531, #31887 ) ;
#147612=EDGE_CURVE ( 'NONE', #122157, #27947, #61062, .T. ) ;
#147708=AXIS2_PLACEMENT_3D ( 'NONE', #129254, #158610, #161606 ) ;
#147804=DIRECTION ( 'NONE',  ( 0.000000000000000000, -0.8164965809277221487, 0.5773502691896313932 ) ) ;
#147987=ORIENTED_EDGE ( 'NONE', *, *, #175772, .F. ) ;
#147995=CARTESIAN_POINT ( 'NONE',  ( -18.96320343559654731, -23.46320343559632704, 8.889087296526001936 ) ) ;
#148051=CARTESIAN_POINT ( 'NONE',  ( -7.500000000000000888, -1.380023386739105851, 5.672916605552547509 ) ) ;
#148103=CIRCLE ( 'NONE', #164280, 5.000000000000000888 ) ;
#148170=CARTESIAN_POINT ( 'NONE',  ( 20.96320343559639454, -21.46320343559646560, 5.353553390593270400 ) ) ;
#148348=ORIENTED_EDGE ( 'NONE', *, *, #25449, .T. ) ;
#148535=LINE ( 'NONE', #10026, #44451 ) ;
#148569=CARTESIAN_POINT ( 'NONE',  ( 7.052343178074640839, -2.552343178074650609, 8.889087296526001936 ) ) ;
#148648=CIRCLE ( 'NONE', #42144, 5.000000000000000000 ) ;
#148657=DIRECTION ( 'NONE',  ( -0.000000000000000000, 0.7071067811865467956, 0.7071067811865483499 ) ) ;
#148707=CARTESIAN_POINT ( 'NONE',  ( -20.96320343559653665, -21.46320343559631638, 4.646446609406719830 ) ) ;
#148914=( BOUNDED_CURVE ( )  B_SPLINE_CURVE ( 3, ( #51619, #128448, #70794, #176988 ),
 .UNSPECIFIED., .F., .F. ) 
 B_SPLINE_CURVE_WITH_KNOTS ( ( 4, 4 ),
 ( 1.025647941782810602, 2.008945357379067431 ),
 .UNSPECIFIED. ) 
 CURVE ( )  GEOMETRIC_REPRESENTATION_ITEM ( )  RATIONAL_B_SPLINE_CURVE ( ( 1.000000000000000000, 0.9210371567966662010, 0.9210371567966662010, 1.000000000000000000 ) ) 
 REPRESENTATION_ITEM ( '' )  );
#148967=DIRECTION ( 'NONE',  ( 0.000000000000000000, -0.7071067811865483499, -0.7071067811865465735 ) ) ;
#149007=ADVANCED_FACE ( 'NONE', ( #39687 ), #184183, .T. ) ;
#149135=EDGE_CURVE ( 'NONE', #64689, #175496, #168989, .T. ) ;
#149423=CARTESIAN_POINT ( 'NONE',  ( -3.889087296526137383, -34.99999999999999289, 1.818019484660534424 ) ) ;
#149468=DIRECTION ( 'NONE',  ( 0.4999999999999933387, -0.5000000000000055511, 0.7071067811865483499 ) ) ;
#149478=LINE ( 'NONE', #86800, #111514 ) ;
#149561=DIRECTION ( 'NONE',  ( 0.8164965809277262565, 0.000000000000000000, 0.5773502691896253980 ) ) ;
#149674=FACE_OUTER_BOUND ( 'NONE', #10721, .T. ) ;
#149760=ADVANCED_FACE ( 'NONE', ( #140646 ), #188168, .F. ) ;
#149803=AXIS2_PLACEMENT_3D ( 'NONE', #126704, #51867, #175221 ) ;
#149829=DIRECTION ( 'NONE',  ( -0.000000000000000000, -0.000000000000000000, 1.000000000000000000 ) ) ;
#149866=DIRECTION ( 'NONE',  ( -0.5000000000000002220, -0.4999999999999985567, 0.7071067811865484609 ) ) ;
#150008=DIRECTION ( 'NONE',  ( 0.000000000000000000, -0.8164965809277252573, 0.5773502691896267303 ) ) ;
#150034=EDGE_CURVE ( 'NONE', #129810, #20570, #135922, .T. ) ;
#150207=AXIS2_PLACEMENT_3D ( 'NONE', #125266, #186964, #2908 ) ;
#150234=ORIENTED_EDGE ( 'NONE', *, *, #28043, .T. ) ;
#150311=EDGE_LOOP ( 'NONE', ( #61198, #5983, #12043, #7479 ) ) ;
#150721=CARTESIAN_POINT ( 'NONE',  ( 0.000000000000000000, 0.000000000000000000, 10.00000000000000000 ) ) ;
#150771=( LENGTH_UNIT ( ) NAMED_UNIT ( * ) SI_UNIT ( .MILLI., .METRE. ) );
#150848=VECTOR ( 'NONE', #34781, 1000.000000000000000 ) ;
#150874=DIRECTION ( 'NONE',  ( 0.8164965809277262565, 0.000000000000000000, 0.5773502691896253980 ) ) ;
#150915=EDGE_CURVE ( 'NONE', #50238, #196966, #148914, .T. ) ;
#151000=FACE_OUTER_BOUND ( 'NONE', #115887, .T. ) ;
#151076=DIRECTION ( 'NONE',  ( 0.8164965809277259234, 0.000000000000000000, 0.5773502691896259531 ) ) ;
#151929=CARTESIAN_POINT ( 'NONE',  ( 20.96320343559639099, -21.46320343559646915, 5.353553390593268624 ) ) ;
#152060=DIRECTION ( 'NONE',  ( 0.000000000000000000, 0.000000000000000000, -1.000000000000000000 ) ) ;
#152161=VERTEX_POINT ( 'NONE', #127807 ) ;
#152294=EDGE_CURVE ( 'NONE', #6681, #96881, #70148, .T. ) ;
#152327=VERTEX_POINT ( 'NONE', #147995 ) ;
#152662=FACE_OUTER_BOUND ( 'NONE', #159848, .T. ) ;
#152730=PRESENTATION_STYLE_ASSIGNMENT (( #103262 ) ) ;
#152909=CARTESIAN_POINT ( 'NONE',  ( -3.424326230466362198, -6.677994727576205491, 1.353258418600858493 ) ) ;
#152912=CYLINDRICAL_SURFACE ( 'NONE', #73511, 5.000000000000000888 ) ;
#152935=ORIENTED_EDGE ( 'NONE', *, *, #96176, .T. ) ;
#153204=AXIS2_PLACEMENT_3D ( 'NONE', #149423, #147431, #192938 ) ;
#153261=( BOUNDED_CURVE ( )  B_SPLINE_CURVE ( 3, ( #45082, #168414, #14739, #76400 ),
 .UNSPECIFIED., .F., .T. ) 
 B_SPLINE_CURVE_WITH_KNOTS ( ( 4, 4 ),
 ( 2.008945357379068319, 2.115944711806983847 ),
 .UNSPECIFIED. ) 
 CURVE ( )  GEOMETRIC_REPRESENTATION_ITEM ( )  RATIONAL_B_SPLINE_CURVE ( ( 1.000000000000000000, 0.9990461557208837329, 0.9990461557208837329, 1.000000000000000000 ) ) 
 REPRESENTATION_ITEM ( '' )  );
#153279=DIRECTION ( 'NONE',  ( 0.000000000000000000, -0.8164965809277251463, 0.5773502691896268413 ) ) ;
#153351=VECTOR ( 'NONE', #47436, 1000.000000000000000 ) ;
#153380=AXIS2_PLACEMENT_3D ( 'NONE', #1367, #63046, #183432 ) ;
#153385=CIRCLE ( 'NONE', #108206, 5.000000000000000000 ) ;
#153392=ADVANCED_FACE ( 'NONE', ( #4970 ), #30610, .T. ) ;
#153625=FACE_OUTER_BOUND ( 'NONE', #103203, .T. ) ;
#153790=EDGE_LOOP ( 'NONE', ( #45028, #24590, #84223, #42569 ) ) ;
#153939=VERTEX_POINT ( 'NONE', #39319 ) ;
#154057=DIRECTION ( 'NONE',  ( -0.000000000000000000, -0.000000000000000000, -1.000000000000000000 ) ) ;
#154058=LINE ( 'NONE', #15553, #29290 ) ;
#154133=EDGE_CURVE ( 'NONE', #114656, #86241, #11932, .T. ) ;
#154255=LINE ( 'NONE', #21707, #15282 ) ;
#154359=ORIENTED_EDGE ( 'NONE', *, *, #87117, .F. ) ;
#154672=CIRCLE ( 'NONE', #6136, 7.500000000000000000 ) ;
#154906=CARTESIAN_POINT ( 'NONE',  ( -3.889087296526037463, -6.412877669190318208, 1.818019484660534424 ) ) ;
#154940=DIRECTION ( 'NONE',  ( 0.8164965809277259234, 0.000000000000000000, 0.5773502691896259531 ) ) ;
#155322=EDGE_CURVE ( 'NONE', #125536, #56096, #162422, .T. ) ;
#155357=ORIENTED_EDGE ( 'NONE', *, *, #162596, .T. ) ;
#155495=DIRECTION ( 'NONE',  ( 1.000000000000000000, 0.000000000000000000, -0.000000000000000000 ) ) ;
#155617=CARTESIAN_POINT ( 'NONE',  ( -6.551653823223136719, -3.660253528765625486, 8.410814283099844246 ) ) ;
#155634=( BOUNDED_CURVE ( )  B_SPLINE_CURVE ( 3, ( #148569, #30940, #177915, #56557 ),
 .UNSPECIFIED., .F., .T. ) 
 B_SPLINE_CURVE_WITH_KNOTS ( ( 4, 4 ),
 ( 5.150538010968860547, 5.257537365396776075 ),
 .UNSPECIFIED. ) 
 CURVE ( )  GEOMETRIC_REPRESENTATION_ITEM ( )  RATIONAL_B_SPLINE_CURVE ( ( 1.000000000000000000, 0.9990461557208837329, 0.9990461557208837329, 1.000000000000000000 ) ) 
 REPRESENTATION_ITEM ( '' )  );
#155808=CARTESIAN_POINT ( 'NONE',  ( 21.46320343559639454, -20.96320343559646915, 4.646446609406721606 ) ) ;
#156050=EDGE_LOOP ( 'NONE', ( #155357, #24008, #67610, #145393, #42287, #173879 ) ) ;
#156137=CARTESIAN_POINT ( 'NONE',  ( 3.181980515339834614, 34.99999999999997158, 1.110912703473986074 ) ) ;
#156226=CARTESIAN_POINT ( 'NONE',  ( -6.674792076160493082, 4.273745901508186229, 5.990689250852173409 ) ) ;
#156324=CARTESIAN_POINT ( 'NONE',  ( -1.784589286804288299, -7.284589286804248331, 8.181980515339454030 ) ) ;
#156408=CIRCLE ( 'NONE', #159711, 4.500000000000000000 ) ;
#156416=VECTOR ( 'NONE', #20191, 1000.000000000000114 ) ;
#156430=DIRECTION ( 'NONE',  ( 0.000000000000000000, -0.7071067811865483499, 0.7071067811865467956 ) ) ;
#156567=AXIS2_PLACEMENT_3D ( 'NONE', #117622, #102453, #148967 ) ;
#156674=CYLINDRICAL_SURFACE ( 'NONE', #72888, 5.000000000000000888 ) ;
#156982=ORIENTED_EDGE ( 'NONE', *, *, #20248, .F. ) ;
#156994=EDGE_CURVE ( 'NONE', #195827, #132628, #198659, .T. ) ;
#157010=VECTOR ( 'NONE', #41696, 1000.000000000000114 ) ;
#157056=DIRECTION ( 'NONE',  ( 0.000000000000000000, -0.7071067811865485719, 0.7071067811865465735 ) ) ;
#157107=CYLINDRICAL_SURFACE ( 'NONE', #1624, 5.000000000000000888 ) ;
#157295=ORIENTED_EDGE ( 'NONE', *, *, #57355, .F. ) ;
#157313=AXIS2_PLACEMENT_3D ( 'NONE', #78641, #31165, #155495 ) ;
#157346=ORIENTED_EDGE ( 'NONE', *, *, #42622, .T. ) ;
#157461=EDGE_CURVE ( 'NONE', #172390, #26894, #111592, .T. ) ;
#157811=ADVANCED_FACE ( 'NONE', ( #33763 ), #157107, .T. ) ;
#157949=VERTEX_POINT ( 'NONE', #65087 ) ;
#157970=ORIENTED_EDGE ( 'NONE', *, *, #181979, .F. ) ;
#158042=EDGE_CURVE ( 'NONE', #152327, #17363, #50924, .T. ) ;
#158147=AXIS2_PLACEMENT_3D ( 'NONE', #50513, #54491, #66660 ) ;
#158220=CARTESIAN_POINT ( 'NONE',  ( -21.46320343559653665, -20.96320343559631638, 5.353553390593268624 ) ) ;
#158445=CARTESIAN_POINT ( 'NONE',  ( 18.46320343559638388, -23.96320343559646915, 1.818019484660534424 ) ) ;
#158610=DIRECTION ( 'NONE',  ( -0.5000000000000049960, -0.4999999999999962252, 0.7071067811865466846 ) ) ;
#159190=VERTEX_POINT ( 'NONE', #139695 ) ;
#159372=ADVANCED_FACE ( 'NONE', ( #112355 ), #97163, .T. ) ;
#159519=CARTESIAN_POINT ( 'NONE',  ( 7.500000000000001776, -1.104226503365433709, 3.188666715448014610 ) ) ;
#159598=FACE_OUTER_BOUND ( 'NONE', #101482, .T. ) ;
#159608=CIRCLE ( 'NONE', #185466, 5.000000000000000000 ) ;
#159665=VECTOR ( 'NONE', #4050, 1000.000000000000000 ) ;
#159692=VECTOR ( 'NONE', #59561, 1000.000000000000000 ) ;
#159693=ORIENTED_EDGE ( 'NONE', *, *, #158042, .F. ) ;
#159711=AXIS2_PLACEMENT_3D ( 'NONE', #25474, #29437, #60742 ) ;
#159748=ADVANCED_FACE ( 'NONE', ( #79023 ), #140698, .T. ) ;
#159848=EDGE_LOOP ( 'NONE', ( #49938, #86775, #62912, #35341 ) ) ;
#159869=ORIENTED_EDGE ( 'NONE', *, *, #147612, .F. ) ;
#159891=CARTESIAN_POINT ( 'NONE',  ( 6.412877669190335972, -3.889087296526014814, 1.818019484660534424 ) ) ;
#160091=AXIS2_PLACEMENT_3D ( 'NONE', #166294, #74277, #120749 ) ;
#160115=( BOUNDED_CURVE ( )  B_SPLINE_CURVE ( 3, ( #142206, #125061, #36019, #93717 ),
 .UNSPECIFIED., .F., .F. ) 
 B_SPLINE_CURVE_WITH_KNOTS ( ( 4, 4 ),
 ( 1.025647941782810824, 2.008945357379067875 ),
 .UNSPECIFIED. ) 
 CURVE ( )  GEOMETRIC_REPRESENTATION_ITEM ( )  RATIONAL_B_SPLINE_CURVE ( ( 1.000000000000000000, 0.9210371567966660900, 0.9210371567966660900, 1.000000000000000000 ) ) 
 REPRESENTATION_ITEM ( '' )  );
#160243=DIRECTION ( 'NONE',  ( 0.000000000000000000, 0.7071067811865467956, -0.7071067811865483499 ) ) ;
#160293=EDGE_CURVE ( 'NONE', #97685, #123075, #45553, .T. ) ;
#160375=CARTESIAN_POINT ( 'NONE',  ( -3.889087296525950421, 6.412877669190374164, 8.181980515339454030 ) ) ;
#160782=COLOUR_RGB ( '', 0.09019608, 0.27058824, 0.51372549) ;
#160889=CARTESIAN_POINT ( 'NONE',  ( -7.052343178074620411, 2.552343178074692354, 8.889087296526001936 ) ) ;
#161086=ORIENTED_EDGE ( 'NONE', *, *, #167192, .F. ) ;
#161122=FACE_OUTER_BOUND ( 'NONE', #97992, .T. ) ;
#161139=UNCERTAINTY_MEASURE_WITH_UNIT (LENGTH_MEASURE( 1.000000000000000082E-05 ), #150771, 'distance_accuracy_value', 'NONE');
#161208=CARTESIAN_POINT ( 'NONE',  ( -27.49873734152928151, -21.99873734152901861, 1.818019484660534424 ) ) ;
#161468=EDGE_CURVE ( 'NONE', #110145, #93013, #178213, .T. ) ;
#161606=DIRECTION ( 'NONE',  ( 0.8164965809277229258, 0.000000000000000000, 0.5773502691896299499 ) ) ;
#161662=ADVANCED_FACE ( 'NONE', ( #146857 ), #194382, .F. ) ;
#161685=APPLICATION_CONTEXT ( 'automotive_design' ) ;
#161687=DIRECTION ( 'NONE',  ( -2.775557561562891351E-15, -0.8164965809277244801, -0.5773502691896280625 ) ) ;
#161725=DIRECTION ( 'NONE',  ( 0.8164965809277261455, 0.000000000000000000, 0.5773502691896257311 ) ) ;
#161882=CARTESIAN_POINT ( 'NONE',  ( -18.46320343559654731, -23.96320343559633059, 8.181980515339454030 ) ) ;
#161996=CARTESIAN_POINT ( 'NONE',  ( -21.46320343559624533, 20.96320343559661836, 4.646446609406719830 ) ) ;
#162125=CARTESIAN_POINT ( 'NONE',  ( 0.000000000000000000, 0.000000000000000000, 10.00000000000000000 ) ) ;
#162170=CARTESIAN_POINT ( 'NONE',  ( -30.00000000000000355, 3.889087296526014814, 1.818019484660534424 ) ) ;
#162209=CARTESIAN_POINT ( 'NONE',  ( -7.128481858827109718, -2.709097808555398945, 7.001991027368838161 ) ) ;
#162333=EDGE_CURVE ( 'NONE', #199879, #17363, #177264, .T. ) ;
#162351=DIRECTION ( 'NONE',  ( -0.5000000000000037748, -0.4999999999999949485, -0.7071067811865484609 ) ) ;
#162422=LINE ( 'NONE', #5740, #53288 ) ;
#162483=ADVANCED_FACE ( 'NONE', ( #198347 ), #31479, .T. ) ;
#162493=CIRCLE ( 'NONE', #55984, 5.000000000000000888 ) ;
#162596=EDGE_CURVE ( 'NONE', #28437, #153939, #170007, .T. ) ;
#162728=CARTESIAN_POINT ( 'NONE',  ( -3.181980515339492221, -6.791538853603052317, 1.110912703473986074 ) ) ;
#162830=CARTESIAN_POINT ( 'NONE',  ( -20.96320343559624177, 21.46320343559661126, 5.353553390593267736 ) ) ;
#162849=ORIENTED_EDGE ( 'NONE', *, *, #41288, .T. ) ;
#162885=CARTESIAN_POINT ( 'NONE',  ( -30.00000000000000355, -0.3535533905932755627, 4.646446609406720718 ) ) ;
#162957=CARTESIAN_POINT ( 'NONE',  ( 22.49873734152949112, 26.99873734152889782, 8.889087296526001936 ) ) ;
#162961=ORIENTED_EDGE ( 'NONE', *, *, #184979, .T. ) ;
#163134=ORIENTED_EDGE ( 'NONE', *, *, #109494, .F. ) ;
#163138=AXIS2_PLACEMENT_3D ( 'NONE', #174046, #5159, #188220 ) ;
#163276=EDGE_LOOP ( 'NONE', ( #100191, #17909, #71612, #179705, #90460, #140363 ) ) ;
#163296=CIRCLE ( 'NONE', #160091, 7.500000000000000000 ) ;
#163352=ORIENTED_EDGE ( 'NONE', *, *, #12432, .T. ) ;
#163678=CYLINDRICAL_SURFACE ( 'NONE', #23886, 5.000000000000000888 ) ;
#163707=ORIENTED_EDGE ( 'NONE', *, *, #100813, .T. ) ;
#163827=CARTESIAN_POINT ( 'NONE',  ( -30.00000000000000355, 3.181980515339468241, 1.110912703473986074 ) ) ;
#164172=PLANE ( 'NONE',  #47247 ) ;
#164280=AXIS2_PLACEMENT_3D ( 'NONE', #121905, #138076, #169399 ) ;
#164900=DIRECTION ( 'NONE',  ( -0.000000000000000000, -0.7071067811865466846, -0.7071067811865484609 ) ) ;
#165029=CARTESIAN_POINT ( 'NONE',  ( 4.962140900324507164, 6.180203150055796790, 6.568406857878971827 ) ) ;
#165093=ORIENTED_EDGE ( 'NONE', *, *, #126396, .F. ) ;
#165110=ADVANCED_FACE ( 'NONE', ( #36850 ), #35864, .T. ) ;
#165127=DIRECTION ( 'NONE',  ( -0.4999999999999967248, 0.5000000000000019984, 0.7071067811865484609 ) ) ;
#165298=LINE ( 'NONE', #26791, #31316 ) ;
#165314=AXIS2_PLACEMENT_3D ( 'NONE', #36600, #51780, #113440 ) ;
#165429=VERTEX_POINT ( 'NONE', #144035 ) ;
#165696=EDGE_CURVE ( 'NONE', #45713, #159190, #99526, .T. ) ;
#165770=VECTOR ( 'NONE', #29707, 1000.000000000000000 ) ;
#166041=FACE_OUTER_BOUND ( 'NONE', #13686, .T. ) ;
#166092=CIRCLE ( 'NONE', #143521, 5.000000000000000888 ) ;
#166140=CARTESIAN_POINT ( 'NONE',  ( 35.00000000000000000, -3.889087296526014814, 1.818019484660534424 ) ) ;
#166294=CARTESIAN_POINT ( 'NONE',  ( 0.000000000000000000, 0.000000000000000000, 10.00000000000000000 ) ) ;
#166341=DIRECTION ( 'NONE',  ( -0.5000000000000002220, -0.4999999999999985012, 0.7071067811865483499 ) ) ;
#166352=ORIENTED_EDGE ( 'NONE', *, *, #93254, .T. ) ;
#166399=VERTEX_POINT ( 'NONE', #28321 ) ;
#166525=ORIENTED_EDGE ( 'NONE', *, *, #128355, .T. ) ;
#166675=DIRECTION ( 'NONE',  ( -0.7071067811865467956, 7.406550393246788537E-15, -0.7071067811865483499 ) ) ;
#166707=VERTEX_POINT ( 'NONE', #163827 ) ;
#166757=ORIENTED_EDGE ( 'NONE', *, *, #55, .F. ) ;
#166940=ORIENTED_EDGE ( 'NONE', *, *, #101975, .F. ) ;
#167007=FACE_BOUND ( 'NONE', #99220, .T. ) ;
#167033=DIRECTION ( 'NONE',  ( 0.7071067811865466846, -7.406550393246786959E-15, 0.7071067811865484609 ) ) ;
#167042=AXIS2_PLACEMENT_3D ( 'NONE', #3693, #83516, #50224 ) ;
#167174=EDGE_LOOP ( 'NONE', ( #122164, #108458, #125644, #70918, #105481, #64857 ) ) ;
#167192=EDGE_CURVE ( 'NONE', #166707, #178298, #56646, .T. ) ;
#167284=VECTOR ( 'NONE', #117681, 1000.000000000000000 ) ;
#167383=ADVANCED_FACE ( 'NONE', ( #152662 ), #43515, .T. ) ;
#167384=ORIENTED_EDGE ( 'NONE', *, *, #177829, .T. ) ;
#167487=EDGE_CURVE ( 'NONE', #120670, #116832, #53222, .T. ) ;
#167515=DIRECTION ( 'NONE',  ( 0.000000000000000000, 0.8164965809277232589, 0.5773502691896297279 ) ) ;
#167752=( LENGTH_UNIT ( ) NAMED_UNIT ( * ) SI_UNIT ( .MILLI., .METRE. ) );
#167974=AXIS2_PLACEMENT_3D ( 'NONE', #7567, #69253, #51096 ) ;
#168234=DIRECTION ( 'NONE',  ( -1.000000000000000000, 0.000000000000000000, 0.000000000000000000 ) ) ;
#168301=ORIENTED_EDGE ( 'NONE', *, *, #87134, .F. ) ;
#168414=CARTESIAN_POINT ( 'NONE',  ( -7.143419655154886527, -2.300691058039395553, 1.353258418600862045 ) ) ;
#168500=EDGE_CURVE ( 'NONE', #120670, #58517, #26096, .T. ) ;
#168680=CARTESIAN_POINT ( 'NONE',  ( -35.00000000000000000, 0.3535533905932707888, 5.353553390593270400 ) ) ;
#168721=EDGE_CURVE ( 'NONE', #175496, #129810, #165298, .T. ) ;
#168850=LINE ( 'NONE', #139505, #33704 ) ;
#168989=LINE ( 'NONE', #43684, #124584 ) ;
#169108=CARTESIAN_POINT ( 'NONE',  ( 1.784589286804253661, -7.284589286804279418, 1.818019484660534424 ) ) ;
#169156=EDGE_LOOP ( 'NONE', ( #8055, #59666, #163352, #39044, #104022, #81982 ) ) ;
#169236=DIRECTION ( 'NONE',  ( 0.7071067811865467956, -7.406550393246788537E-15, 0.7071067811865483499 ) ) ;
#169373=ORIENTED_EDGE ( 'NONE', *, *, #161468, .F. ) ;
#169399=DIRECTION ( 'NONE',  ( 0.000000000000000000, -0.7071067811865483499, -0.7071067811865465735 ) ) ;
#169707=AXIS2_PLACEMENT_3D ( 'NONE', #24399, #51714, #21379 ) ;
#169808=ORIENTED_EDGE ( 'NONE', *, *, #167487, .F. ) ;
#169925=DIRECTION ( 'NONE',  ( 1.000000000000000000, 0.000000000000000000, 0.000000000000000000 ) ) ;
#170007=CIRCLE ( 'NONE', #79512, 4.999999999999998224 ) ;
#170048=ORIENTED_EDGE ( 'NONE', *, *, #36780, .F. ) ;
#170135=EDGE_LOOP ( 'NONE', ( #27596, #194316, #31085, #173370 ) ) ;
#170160=ORIENTED_EDGE ( 'NONE', *, *, #90984, .T. ) ;
#170165=ORIENTED_EDGE ( 'NONE', *, *, #139917, .T. ) ;
#170664=ORIENTED_EDGE ( 'NONE', *, *, #27260, .T. ) ;
#170916=EDGE_CURVE ( 'NONE', #52906, #58517, #184913, .T. ) ;
#171004=VECTOR ( 'NONE', #143354, 1000.000000000000114 ) ;
#171113=VECTOR ( 'NONE', #47620, 1000.000000000000000 ) ;
#171120=ADVANCED_FACE ( 'NONE', ( #200017, #93815 ), #139323, .F. ) ;
#171196=CYLINDRICAL_SURFACE ( 'NONE', #104903, 4.500000000000000000 ) ;
#171287=ORIENTED_EDGE ( 'NONE', *, *, #17418, .T. ) ;
#171715=VERTEX_POINT ( 'NONE', #29584 ) ;
#171733=CARTESIAN_POINT ( 'NONE',  ( -21.46320343559653665, -25.04568634023494056, 8.240304736541400388 ) ) ;
#171952=EDGE_CURVE ( 'NONE', #85047, #195827, #92774, .T. ) ;
#172095=AXIS2_PLACEMENT_3D ( 'NONE', #31687, #107511, #139833 ) ;
#172390=VERTEX_POINT ( 'NONE', #84590 ) ;
#172493=EDGE_CURVE ( 'NONE', #115498, #58678, #113927, .T. ) ;
#172548=DIRECTION ( 'NONE',  ( -0.4999999999999967248, 0.5000000000000019984, 0.7071067811865484609 ) ) ;
#172681=VECTOR ( 'NONE', #22226, 1000.000000000000000 ) ;
#172755=( BOUNDED_CURVE ( )  B_SPLINE_CURVE ( 3, ( #88787, #118141, #13931, #71629 ),
 .UNSPECIFIED., .F., .T. ) 
 B_SPLINE_CURVE_WITH_KNOTS ( ( 4, 4 ),
 ( 2.008945357379066987, 2.115944711806982070 ),
 .UNSPECIFIED. ) 
 CURVE ( )  GEOMETRIC_REPRESENTATION_ITEM ( )  RATIONAL_B_SPLINE_CURVE ( ( 1.000000000000000000, 0.9990461557208837329, 0.9990461557208837329, 1.000000000000000000 ) ) 
 REPRESENTATION_ITEM ( '' )  );
#172787=CARTESIAN_POINT ( 'NONE',  ( -6.412877669190332419, -3.889087296526017479, 8.181980515339454030 ) ) ;
#172822=ORIENTED_EDGE ( 'NONE', *, *, #162596, .F. ) ;
#172837=DIRECTION ( 'NONE',  ( 0.000000000000000000, 0.000000000000000000, 1.000000000000000000 ) ) ;
#173150=EDGE_LOOP ( 'NONE', ( #159869, #61406, #176901, #188268 ) ) ;
#173307=CARTESIAN_POINT ( 'NONE',  ( 7.500000000000000000, 9.184850993605147944E-16, 10.00000000000000000 ) ) ;
#173343=CIRCLE ( 'NONE', #86167, 5.000000000000000888 ) ;
#173370=ORIENTED_EDGE ( 'NONE', *, *, #1347, .F. ) ;
#173397=LINE ( 'NONE', #33881, #60900 ) ;
#173459=FACE_OUTER_BOUND ( 'NONE', #69902, .T. ) ;
#173518=EDGE_CURVE ( 'NONE', #166707, #46039, #193806, .T. ) ;
#173548=CARTESIAN_POINT ( 'NONE',  ( -30.00000000000000355, -0.3535533905932735643, 4.646446609406718942 ) ) ;
#173582=ORIENTED_EDGE ( 'NONE', *, *, #17418, .F. ) ;
#173649=AXIS2_PLACEMENT_3D ( 'NONE', #94749, #156430, #17930 ) ;
#173824=ORIENTED_EDGE ( 'NONE', *, *, #94772, .T. ) ;
#173854=DIRECTION ( 'NONE',  ( 0.000000000000000000, 0.7071067811865483499, -0.7071067811865467956 ) ) ;
#173879=ORIENTED_EDGE ( 'NONE', *, *, #174237, .F. ) ;
#173900=CARTESIAN_POINT ( 'NONE',  ( -23.96320343559652599, -18.46320343559629862, 1.818019484660532648 ) ) ;
#173940=( BOUNDED_CURVE ( )  B_SPLINE_CURVE ( 3, ( #64222, #50048, #156226, #142039 ),
 .UNSPECIFIED., .F., .F. ) 
 B_SPLINE_CURVE_WITH_KNOTS ( ( 4, 4 ),
 ( 1.132647296210726351, 2.115944711806983403 ),
 .UNSPECIFIED. ) 
 CURVE ( )  GEOMETRIC_REPRESENTATION_ITEM ( )  RATIONAL_B_SPLINE_CURVE ( ( 1.000000000000000000, 0.9210371567966660900, 0.9210371567966660900, 1.000000000000000000 ) ) 
 REPRESENTATION_ITEM ( '' )  );
#174046=CARTESIAN_POINT ( 'NONE',  ( 21.46320343559639099, -20.96320343559646915, 4.646446609406719830 ) ) ;
#174088=CARTESIAN_POINT ( 'NONE',  ( 3.889087296525994830, -6.412877669190346630, 8.181980515339454030 ) ) ;
#174183=CARTESIAN_POINT ( 'NONE',  ( 0.000000000000000000, 0.000000000000000000, 0.000000000000000000 ) ) ;
#174237=EDGE_CURVE ( 'NONE', #28437, #123075, #154255, .T. ) ;
#174324=CARTESIAN_POINT ( 'NONE',  ( -7.220908937439997288, 2.044528755335752734, 8.410814283099849575 ) ) ;
#174543=DIRECTION ( 'NONE',  ( 0.000000000000000000, -0.7071067811865467956, -0.7071067811865483499 ) ) ;
#174803=ORIENTED_EDGE ( 'NONE', *, *, #143563, .F. ) ;
#174809=CARTESIAN_POINT ( 'NONE',  ( -3.889087296526137383, -34.99999999999999289, 1.818019484660534424 ) ) ;
#175109=EDGE_LOOP ( 'NONE', ( #54526, #23455, #111587, #161086 ) ) ;
#175221=DIRECTION ( 'NONE',  ( 1.000000000000000000, 0.000000000000000000, 0.000000000000000000 ) ) ;
#175395=ORIENTED_EDGE ( 'NONE', *, *, #42622, .F. ) ;
#175416=DIRECTION ( 'NONE',  ( 0.000000000000000000, 0.000000000000000000, -1.000000000000000000 ) ) ;
#175439=PLANE ( 'NONE',  #167974 ) ;
#175496=VERTEX_POINT ( 'NONE', #179378 ) ;
#175772=EDGE_CURVE ( 'NONE', #48994, #97685, #137564, .T. ) ;
#175795=CIRCLE ( 'NONE', #114428, 4.999999999999998224 ) ;
#176579=CARTESIAN_POINT ( 'NONE',  ( 7.500000000000000000, 9.184850993605147944E-16, 4.292893218813446765 ) ) ;
#176901=ORIENTED_EDGE ( 'NONE', *, *, #58459, .F. ) ;
#176988=CARTESIAN_POINT ( 'NONE',  ( 3.181980515339446924, -6.791538853603077186, 8.889087296526001936 ) ) ;
#177083=CARTESIAN_POINT ( 'NONE',  ( -6.791538853603066528, -3.181980515339470905, 8.889087296526001936 ) ) ;
#177264=( BOUNDED_CURVE ( )  B_SPLINE_CURVE ( 3, ( #56862, #105337, #59821, #77964 ),
 .UNSPECIFIED., .F., .T. ) 
 B_SPLINE_CURVE_WITH_KNOTS ( ( 4, 4 ),
 ( 1.025647941782809491, 2.008945357379068319 ),
 .UNSPECIFIED. ) 
 CURVE ( )  GEOMETRIC_REPRESENTATION_ITEM ( )  RATIONAL_B_SPLINE_CURVE ( ( 1.000000000000000000, 0.9210371567966657569, 0.9210371567966657569, 1.000000000000000000 ) ) 
 REPRESENTATION_ITEM ( '' )  );
#177317=FACE_OUTER_BOUND ( 'NONE', #13016, .T. ) ;
#177321=DIRECTION ( 'NONE',  ( 0.000000000000000000, 0.7071067811865466846, 0.7071067811865484609 ) ) ;
#177402=CARTESIAN_POINT ( 'NONE',  ( -7.500000000000000000, 0.000000000000000000, 4.292893218813445877 ) ) ;
#177515=VERTEX_POINT ( 'NONE', #39349 ) ;
#177531=ORIENTED_EDGE ( 'NONE', *, *, #150034, .T. ) ;
#177829=EDGE_CURVE ( 'NONE', #185456, #114656, #148535, .T. ) ;
#177915=CARTESIAN_POINT ( 'NONE',  ( 7.220908937440010611, -2.044528755335700776, 8.410814283099846023 ) ) ;
#177929=EDGE_LOOP ( 'NONE', ( #112174, #180573, #5451, #68097 ) ) ;
#177959=LINE ( 'NONE', #195126, #122466 ) ;
#178213=LINE ( 'NONE', #117523, #157010 ) ;
#178298=VERTEX_POINT ( 'NONE', #162170 ) ;
#178424=CYLINDRICAL_SURFACE ( 'NONE', #198089, 5.000000000000000000 ) ;
#178636=LINE ( 'NONE', #105765, #91873 ) ;
#178806=ORIENTED_EDGE ( 'NONE', *, *, #110020, .T. ) ;
#178830=ORIENTED_EDGE ( 'NONE', *, *, #14195, .F. ) ;
#178851=CARTESIAN_POINT ( 'NONE',  ( 7.500000000000000000, 9.184850993605147944E-16, 5.707106781186540800 ) ) ;
#178898=ORIENTED_EDGE ( 'NONE', *, *, #16838, .F. ) ;
#178912=CARTESIAN_POINT ( 'NONE',  ( 21.46320343559639099, -20.96320343559646915, 4.646446609406719830 ) ) ;
#179081=ADVANCED_FACE ( 'NONE', ( #59967 ), #11514, .F. ) ;
#179113=ORIENTED_EDGE ( 'NONE', *, *, #170916, .T. ) ;
#179141=AXIS2_PLACEMENT_3D ( 'NONE', #25203, #100001, #161687 ) ;
#179207=ADVANCED_FACE ( 'NONE', ( #104500 ), #24679, .T. ) ;
#179214=VECTOR ( 'NONE', #142848, 1000.000000000000000 ) ;
#179378=CARTESIAN_POINT ( 'NONE',  ( 3.889087296526328785, 29.99999999999996092, 1.818019484660534424 ) ) ;
#179632=EDGE_CURVE ( 'NONE', #196966, #41517, #73924, .T. ) ;
#179705=ORIENTED_EDGE ( 'NONE', *, *, #187016, .T. ) ;
#179831=CARTESIAN_POINT ( 'NONE',  ( -0.3535533905929611476, 30.00000000000000711, 4.646446609406721606 ) ) ;
#179855=AXIS2_PLACEMENT_3D ( 'NONE', #148707, #42526, #89014 ) ;
#180052=ORIENTED_EDGE ( 'NONE', *, *, #4454, .T. ) ;
#180191=CARTESIAN_POINT ( 'NONE',  ( -1.784589286804288299, -7.284589286804248331, 8.181980515339454030 ) ) ;
#180236=DIRECTION ( 'NONE',  ( 0.7071067811865483499, 0.000000000000000000, -0.7071067811865465735 ) ) ;
#180286=EDGE_LOOP ( 'NONE', ( #39358, #101215, #137261, #115462 ) ) ;
#180335=CARTESIAN_POINT ( 'NONE',  ( -7.500000000000000000, 0.000000000000000000, 5.707106781186540800 ) ) ;
#180340=VERTEX_POINT ( 'NONE', #52658 ) ;
#180557=CARTESIAN_POINT ( 'NONE',  ( 25.04568634023502582, -21.46320343559646560, 8.240304736541396835 ) ) ;
#180573=ORIENTED_EDGE ( 'NONE', *, *, #44361, .T. ) ;
#180658=ORIENTED_EDGE ( 'NONE', *, *, #184085, .F. ) ;
#180825=LINE ( 'NONE', #135311, #4878 ) ;
#180850=CIRCLE ( 'NONE', #158147, 5.000000000000000000 ) ;
#180917=CARTESIAN_POINT ( 'NONE',  ( -21.46320343559624533, 20.96320343559661481, 4.646446609406719830 ) ) ;
#181119=ADVANCED_FACE ( 'NONE', ( #149674 ), #199152, .T. ) ;
#181269=EDGE_LOOP ( 'NONE', ( #92438, #1856, #173824, #70454, #110214 ) ) ;
#181399=CARTESIAN_POINT ( 'NONE',  ( -4.500000000000000000, 5.510910596163088569E-16, 0.000000000000000000 ) ) ;
#181421=CARTESIAN_POINT ( 'NONE',  ( 6.677994727576218814, -3.424326230466335996, 1.353258418600855606 ) ) ;
#181724=ADVANCED_FACE ( 'NONE', ( #35260 ), #80759, .T. ) ;
#181795=VECTOR ( 'NONE', #55576, 1000.000000000000000 ) ;
#181840=CARTESIAN_POINT ( 'NONE',  ( -0.3535533905929588716, 30.00000000000000711, 4.646446609406719830 ) ) ;
#181848=ORIENTED_EDGE ( 'NONE', *, *, #132933, .F. ) ;
#181931=AXIS2_PLACEMENT_3D ( 'NONE', #129876, #50088, #189599 ) ;
#181979=EDGE_CURVE ( 'NONE', #79638, #195827, #188968, .T. ) ;
#182032=CARTESIAN_POINT ( 'NONE',  ( 7.052343178074679031, 2.552343178074557350, 1.110912703473986074 ) ) ;
#182172=LINE ( 'NONE', #45637, #93639 ) ;
#182789=DIRECTION ( 'NONE',  ( 0.8164965809277243691, 0.000000000000000000, -0.5773502691896280625 ) ) ;
#182929=FILL_AREA_STYLE_COLOUR ( '', #160782 ) ;
#183156=EDGE_CURVE ( 'NONE', #42832, #85800, #88744, .T. ) ;
#183167=VECTOR ( 'NONE', #44239, 999.9999999999998863 ) ;
#183432=DIRECTION ( 'NONE',  ( 0.7071067811865483499, 0.000000000000000000, -0.7071067811865465735 ) ) ;
#183469=ORIENTED_EDGE ( 'NONE', *, *, #17615, .T. ) ;
#183693=EDGE_CURVE ( 'NONE', #58678, #93013, #8817, .T. ) ;
#183854=ORIENTED_EDGE ( 'NONE', *, *, #116186, .F. ) ;
#184079=ORIENTED_EDGE ( 'NONE', *, *, #13320, .F. ) ;
#184085=EDGE_CURVE ( 'NONE', #20570, #89709, #107532, .T. ) ;
#184106=DIRECTION ( 'NONE',  ( -1.000000000000000000, 0.000000000000000000, 0.000000000000000000 ) ) ;
#184110=CARTESIAN_POINT ( 'NONE',  ( -35.00000000000000000, -0.3535533905932759513, 4.646446609406721606 ) ) ;
#184183=PLANE ( 'NONE',  #11630 ) ;
#184276=LINE ( 'NONE', #166140, #59872 ) ;
#184297=CARTESIAN_POINT ( 'NONE',  ( 20.96320343559639454, -21.46320343559646560, 5.353553390593268624 ) ) ;
#184417=ORIENTED_EDGE ( 'NONE', *, *, #114488, .T. ) ;
#184434=CARTESIAN_POINT ( 'NONE',  ( -18.96320343559621691, 23.46320343559659705, 1.110912703473986074 ) ) ;
#184645=DIRECTION ( 'NONE',  ( -0.8164965809277229258, 0.000000000000000000, -0.5773502691896299499 ) ) ;
#184763=ORIENTED_EDGE ( 'NONE', *, *, #56725, .F. ) ;
#184811=ORIENTED_EDGE ( 'NONE', *, *, #40219, .T. ) ;
#184843=CARTESIAN_POINT ( 'NONE',  ( 1.784589286804354247, 7.284589286804251884, 8.181980515339454030 ) ) ;
#184866=EDGE_CURVE ( 'NONE', #19226, #723, #173343, .T. ) ;
#184913=( BOUNDED_CURVE ( )  B_SPLINE_CURVE ( 3, ( #32158, #77655, #187843, #184843 ),
 .UNSPECIFIED., .F., .F. ) 
 B_SPLINE_CURVE_WITH_KNOTS ( ( 4, 4 ),
 ( 5.150538010968860547, 5.257537365396775186 ),
 .UNSPECIFIED. ) 
 CURVE ( )  GEOMETRIC_REPRESENTATION_ITEM ( )  RATIONAL_B_SPLINE_CURVE ( ( 1.000000000000000000, 0.9990461557208837329, 0.9990461557208837329, 1.000000000000000000 ) ) 
 REPRESENTATION_ITEM ( '' )  );
#184964=CARTESIAN_POINT ( 'NONE',  ( -6.791538853603066528, -3.181980515339470905, 8.889087296526001936 ) ) ;
#184979=EDGE_CURVE ( 'NONE', #89057, #13627, #40003, .T. ) ;
#185021=CARTESIAN_POINT ( 'NONE',  ( 35.00000000000000000, 0.3535533905932759513, 4.646446609406721606 ) ) ;
#185043=PLANE ( 'NONE',  #32314 ) ;
#185200=CARTESIAN_POINT ( 'NONE',  ( -0.3535533905933764265, -30.00000000000000355, 5.353553390593269512 ) ) ;
#185258=DIRECTION ( 'NONE',  ( 0.000000000000000000, -0.8164965809277232589, -0.5773502691896295058 ) ) ;
#185456=VERTEX_POINT ( 'NONE', #71353 ) ;
#185466=AXIS2_PLACEMENT_3D ( 'NONE', #96057, #80884, #190074 ) ;
#185490=LINE ( 'NONE', #173307, #89193 ) ;
#185673=EDGE_CURVE ( 'NONE', #64689, #157949, #64133, .T. ) ;
#185759=PRODUCT_DEFINITION_SHAPE ( 'NONE', 'NONE',  #115338 ) ;
#185853=EDGE_CURVE ( 'NONE', #23611, #90645, #185490, .T. ) ;
#185997=LINE ( 'NONE', #187007, #128314 ) ;
#186623=AXIS2_PLACEMENT_3D ( 'NONE', #27682, #102503, #135840 ) ;
#186775=ORIENTED_EDGE ( 'NONE', *, *, #8138, .T. ) ;
#186964=DIRECTION ( 'NONE',  ( -0.5000000000000002220, -0.4999999999999985012, 0.7071067811865483499 ) ) ;
#186982=DIRECTION ( 'NONE',  ( 0.000000000000000000, -0.8164965809277233699, -0.5773502691896295058 ) ) ;
#187007=CARTESIAN_POINT ( 'NONE',  ( -35.00000000000000000, 0.3535533905932703447, 5.353553390593268624 ) ) ;
#187016=EDGE_CURVE ( 'NONE', #93013, #152327, #127846, .T. ) ;
#187186=CARTESIAN_POINT ( 'NONE',  ( -0.8613000766923508689, 7.878827036337495926, 6.568406857878970939 ) ) ;
#187232=ORIENTED_EDGE ( 'NONE', *, *, #36811, .F. ) ;
#187646=DIRECTION ( 'NONE',  ( -0.4999999999999967248, 0.5000000000000019984, 0.7071067811865484609 ) ) ;
#187655=ORIENTED_EDGE ( 'NONE', *, *, #129609, .T. ) ;
#187843=CARTESIAN_POINT ( 'NONE',  ( 2.044528755335782044, 7.220908937439987518, 8.410814283099853128 ) ) ;
#188018=FACE_OUTER_BOUND ( 'NONE', #173150, .T. ) ;
#188103=CARTESIAN_POINT ( 'NONE',  ( -3.181980515339104532, 35.00000000000003553, 8.889087296526001936 ) ) ;
#188168=PLANE ( 'NONE',  #130941 ) ;
#188220=DIRECTION ( 'NONE',  ( -0.8164965809277260345, 0.000000000000000000, -0.5773502691896258421 ) ) ;
#188245=CIRCLE ( 'NONE', #165314, 5.000000000000000000 ) ;
#188268=ORIENTED_EDGE ( 'NONE', *, *, #10280, .F. ) ;
#188282=ORIENTED_EDGE ( 'NONE', *, *, #105202, .F. ) ;
#188357=CARTESIAN_POINT ( 'NONE',  ( -24.49873734152929572, -24.99873734152903282, 4.646446609406721606 ) ) ;
#188682=AXIS2_PLACEMENT_3D ( 'NONE', #8687, #174543, #36010 ) ;
#188739=CARTESIAN_POINT ( 'NONE',  ( -1.697796032038645597, 7.741785448087978416, 5.990689250852168968 ) ) ;
#188832=ORIENTED_EDGE ( 'NONE', *, *, #137445, .T. ) ;
#188910=PRODUCT_DEFINITION_FORMATION_WITH_SPECIFIED_SOURCE ( 'ANY', '', #92061, .NOT_KNOWN. ) ;
#188968=LINE ( 'NONE', #50444, #73359 ) ;
#189355=DIRECTION ( 'NONE',  ( 0.000000000000000000, 0.000000000000000000, -1.000000000000000000 ) ) ;
#189500=EDGE_CURVE ( 'NONE', #159190, #37612, #162493, .T. ) ;
#189599=DIRECTION ( 'NONE',  ( -0.7071067811865483499, 0.000000000000000000, -0.7071067811865466846 ) ) ;
#189622=CARTESIAN_POINT ( 'NONE',  ( -23.46320343559626664, 18.96320343559662902, 8.889087296526001936 ) ) ;
#189812=MECHANICAL_DESIGN_GEOMETRIC_PRESENTATION_REPRESENTATION('',(#121967),#54280);
#189868=ORIENTED_EDGE ( 'NONE', *, *, #132933, .T. ) ;
#189925=DIRECTION ( 'NONE',  ( -0.000000000000000000, -0.000000000000000000, -1.000000000000000000 ) ) ;
#189949=CARTESIAN_POINT ( 'NONE',  ( 3.181980515339348337, -35.00000000000001421, 8.889087296526001936 ) ) ;
#190018=CARTESIAN_POINT ( 'NONE',  ( 7.500000000000001776, 1.104226503365437706, 6.811333284551975176 ) ) ;
#190074=DIRECTION ( 'NONE',  ( 0.000000000000000000, -0.7071067811865485719, 0.7071067811865465735 ) ) ;
#190197=ORIENTED_EDGE ( 'NONE', *, *, #133545, .F. ) ;
#190225=( BOUNDED_CURVE ( )  B_SPLINE_CURVE ( 3, ( #23632, #66130, #174324, #115639 ),
 .UNSPECIFIED., .F., .T. ) 
 B_SPLINE_CURVE_WITH_KNOTS ( ( 4, 4 ),
 ( 5.150538010968860547, 5.257537365396776075 ),
 .UNSPECIFIED. ) 
 CURVE ( )  GEOMETRIC_REPRESENTATION_ITEM ( )  RATIONAL_B_SPLINE_CURVE ( ( 1.000000000000000000, 0.9990461557208837329, 0.9990461557208837329, 1.000000000000000000 ) ) 
 REPRESENTATION_ITEM ( '' )  );
#190273=( LENGTH_UNIT ( ) NAMED_UNIT ( * ) SI_UNIT ( .MILLI., .METRE. ) );
#190433=ORIENTED_EDGE ( 'NONE', *, *, #18906, .F. ) ;
#190434=DIRECTION ( 'NONE',  ( 0.000000000000000000, -0.7071067811865467956, 0.7071067811865483499 ) ) ;
#190488=AXIS2_PLACEMENT_3D ( 'NONE', #108290, #108, #16296 ) ;
#190558=CYLINDRICAL_SURFACE ( 'NONE', #49709, 5.000000000000000000 ) ;
#191005=CARTESIAN_POINT ( 'NONE',  ( 7.260022482700429158, 2.182060888568188251, 7.889167669754723278 ) ) ;
#191239=CARTESIAN_POINT ( 'NONE',  ( -3.181980515339492221, -6.791538853603052317, 1.110912703473986074 ) ) ;
#191246=ORIENTED_EDGE ( 'NONE', *, *, #120835, .F. ) ;
#191334=DIRECTION ( 'NONE',  ( 0.000000000000000000, -0.8164965809277251463, 0.5773502691896268413 ) ) ;
#191436=AXIS2_PLACEMENT_3D ( 'NONE', #77182, #137866, #30694 ) ;
#191473=UNCERTAINTY_MEASURE_WITH_UNIT (LENGTH_MEASURE( 1.000000000000000082E-05 ), #167752, 'distance_accuracy_value', 'NONE');
#191542=DIRECTION ( 'NONE',  ( 0.5000000000000037748, 0.4999999999999949485, 0.7071067811865484609 ) ) ;
#191771=ORIENTED_EDGE ( 'NONE', *, *, #1347, .T. ) ;
#191800=VERTEX_POINT ( 'NONE', #116539 ) ;
#191847=VERTEX_POINT ( 'NONE', #101353 ) ;
#191905=ORIENTED_EDGE ( 'NONE', *, *, #41619, .F. ) ;
#192111=LINE ( 'NONE', #102099, #6595 ) ;
#192198=CARTESIAN_POINT ( 'NONE',  ( 2.552343178074615970, -7.052343178074640839, 1.110912703473986074 ) ) ;
#192235=( BOUNDED_CURVE ( )  B_SPLINE_CURVE ( 3, ( #41878, #194560, #42869, #196566 ),
 .UNSPECIFIED., .F., .T. ) 
 B_SPLINE_CURVE_WITH_KNOTS ( ( 4, 4 ),
 ( 1.570796326794896780, 2.115944711806982959 ),
 .UNSPECIFIED. ) 
 CURVE ( )  GEOMETRIC_REPRESENTATION_ITEM ( )  RATIONAL_B_SPLINE_CURVE ( ( 1.000000000000000000, 0.9753873905749756990, 0.9753873905749756990, 1.000000000000000000 ) ) 
 REPRESENTATION_ITEM ( '' )  );
#192429=EDGE_LOOP ( 'NONE', ( #24595, #45804, #86543, #60779 ) ) ;
#192469=PLANE ( 'NONE',  #143465 ) ;
#192481=AXIS2_PLACEMENT_3D ( 'NONE', #99558, #8564, #160243 ) ;
#192482=LINE ( 'NONE', #67128, #33597 ) ;
#192537=AXIS2_PLACEMENT_3D ( 'NONE', #62793, #123466, #1119 ) ;
#192938=DIRECTION ( 'NONE',  ( 0.7071067811865483499, 0.000000000000000000, 0.7071067811865465735 ) ) ;
#192994=DIRECTION ( 'NONE',  ( 1.000000000000000000, -0.000000000000000000, -0.000000000000000000 ) ) ;
#193239=PLANE ( 'NONE',  #169707 ) ;
#193271=AXIS2_PLACEMENT_3D ( 'NONE', #39096, #85589, #58262 ) ;
#193476=PLANE ( 'NONE',  #87267 ) ;
#193497=EDGE_CURVE ( 'NONE', #42657, #50238, #21117, .T. ) ;
#193792=PLANE ( 'NONE',  #193271 ) ;
#193806=LINE ( 'NONE', #87603, #18467 ) ;
#194261=EDGE_LOOP ( 'NONE', ( #127599, #65386, #41751, #78642 ) ) ;
#194316=ORIENTED_EDGE ( 'NONE', *, *, #3105, .F. ) ;
#194382=PLANE ( 'NONE',  #115018 ) ;
#194528=ADVANCED_FACE ( 'NONE', ( #145864 ), #65048, .T. ) ;
#194560=CARTESIAN_POINT ( 'NONE',  ( 7.500000000000000888, 1.380023386739106961, 5.672916605552548397 ) ) ;
#194637=CARTESIAN_POINT ( 'NONE',  ( 6.180203150055914918, 4.962140900324359727, 3.431593142121018847 ) ) ;
#194728=ORIENTED_EDGE ( 'NONE', *, *, #58459, .T. ) ;
#194786=AXIS2_PLACEMENT_3D ( 'NONE', #111748, #175416, #112733 ) ;
#195071=AXIS2_PLACEMENT_3D ( 'NONE', #180917, #87874, #195079 ) ;
#195079=DIRECTION ( 'NONE',  ( -0.8164965809277243691, 0.000000000000000000, 0.5773502691896281735 ) ) ;
#195120=CLOSED_SHELL ( 'NONE', ( #7349, #181119, #153392, #99122, #34450, #39897, #171120, #134165, #109377, #85440, #38588, #157811, #73604, #12967, #64638, #161662, #96947, #59605, #40135, #89114, #149007, #72193, #119923, #33560, #70007, #78559, #121162, #198694, #121823, #104659, #179081, #2575, #165110, #137794, #181724, #149760, #101197, #11219, #162483, #28210, #63977, #114053, #159372, #64613, #113118, #104650, #167383, #105983, #41055, #159748, #108000, #19925, #102571, #179207, #8948, #194528, #113133 ) ) ;
#195126=CARTESIAN_POINT ( 'NONE',  ( 26.99873734152944138, 22.49873734152883387, 1.110912703473986074 ) ) ;
#195127=COLOUR_RGB ( '', 0.09019608, 0.27058824, 0.51372549) ;
#195346=CARTESIAN_POINT ( 'NONE',  ( -6.180203150055883832, -4.962140900324400583, 3.431593142121015294 ) ) ;
#195441=ORIENTED_EDGE ( 'NONE', *, *, #147508, .F. ) ;
#195479=LINE ( 'NONE', #24627, #96257 ) ;
#195489=DIRECTION ( 'NONE',  ( 0.000000000000000000, -0.8164965809277232589, -0.5773502691896295058 ) ) ;
#195510=CARTESIAN_POINT ( 'NONE',  ( -30.00000000000000355, -3.889087296526017479, 8.181980515339454030 ) ) ;
#195689=ORIENTED_EDGE ( 'NONE', *, *, #96176, .F. ) ;
#195827=VERTEX_POINT ( 'NONE', #49980 ) ;
#195876=ORIENTED_EDGE ( 'NONE', *, *, #72094, .T. ) ;
#196167=VECTOR ( 'NONE', #4756, 1000.000000000000000 ) ;
#196169=EDGE_CURVE ( 'NONE', #152161, #37524, #192482, .T. ) ;
#196199=DIRECTION ( 'NONE',  ( 0.8164965809277243691, 0.000000000000000000, -0.5773502691896280625 ) ) ;
#196211=EDGE_CURVE ( 'NONE', #18224, #36918, #190225, .T. ) ;
#196358=ORIENTED_EDGE ( 'NONE', *, *, #72094, .F. ) ;
#196479=CARTESIAN_POINT ( 'NONE',  ( 30.00000000000000355, 0.3535533905932729537, 4.646446609406719830 ) ) ;
#196537=ORIENTED_EDGE ( 'NONE', *, *, #183693, .F. ) ;
#196566=CARTESIAN_POINT ( 'NONE',  ( 6.412877669190332419, 3.889087296526017479, 8.181980515339454030 ) ) ;
#196688=VERTEX_POINT ( 'NONE', #180335 ) ;
#196966=VERTEX_POINT ( 'NONE', #120611 ) ;
#197329=EDGE_CURVE ( 'NONE', #28306, #41517, #52032, .T. ) ;
#197609=EDGE_LOOP ( 'NONE', ( #147987, #180052, #183469, #23431 ) ) ;
#197769=ORIENTED_EDGE ( 'NONE', *, *, #87117, .T. ) ;
#197973=CARTESIAN_POINT ( 'NONE',  ( -3.181980515339399851, 6.791538853603101167, 8.889087296526001936 ) ) ;
#198089=AXIS2_PLACEMENT_3D ( 'NONE', #9572, #28733, #151076 ) ;
#198347=FACE_OUTER_BOUND ( 'NONE', #197609, .T. ) ;
#198408=ORIENTED_EDGE ( 'NONE', *, *, #36310, .T. ) ;
#198438=CARTESIAN_POINT ( 'NONE',  ( -21.46320343559653665, -20.96320343559631638, 5.353553390593267736 ) ) ;
#198466=ORIENTED_EDGE ( 'NONE', *, *, #126710, .T. ) ;
#198500=EDGE_LOOP ( 'NONE', ( #186775, #138073, #11040, #197769, #168301 ) ) ;
#198588=FACE_BOUND ( 'NONE', #153790, .T. ) ;
#198659=CIRCLE ( 'NONE', #50134, 4.999999999999998224 ) ;
#198694=ADVANCED_FACE ( 'NONE', ( #34333 ), #3974, .T. ) ;
#198707=AXIS2_PLACEMENT_3D ( 'NONE', #112223, #5025, #66710 ) ;
#198713=VERTEX_POINT ( 'NONE', #84796 ) ;
#199013=ORIENTED_EDGE ( 'NONE', *, *, #125179, .F. ) ;
#199067=VERTEX_POINT ( 'NONE', #99972 ) ;
#199152=CYLINDRICAL_SURFACE ( 'NONE', #18750, 5.000000000000000000 ) ;
#199222=EDGE_LOOP ( 'NONE', ( #132749, #162849, #128762, #25888 ) ) ;
#199552=CARTESIAN_POINT ( 'NONE',  ( 0.000000000000000000, 0.000000000000000000, -20.00000000000000000 ) ) ;
#199643=ORIENTED_EDGE ( 'NONE', *, *, #173518, .T. ) ;
#199879=VERTEX_POINT ( 'NONE', #114408 ) ;
#199998=CIRCLE ( 'NONE', #64459, 4.500000000000000000 ) ;
#200017=FACE_BOUND ( 'NONE', #135372, .T. ) ;
ENDSEC;
END-ISO-10303-21;
